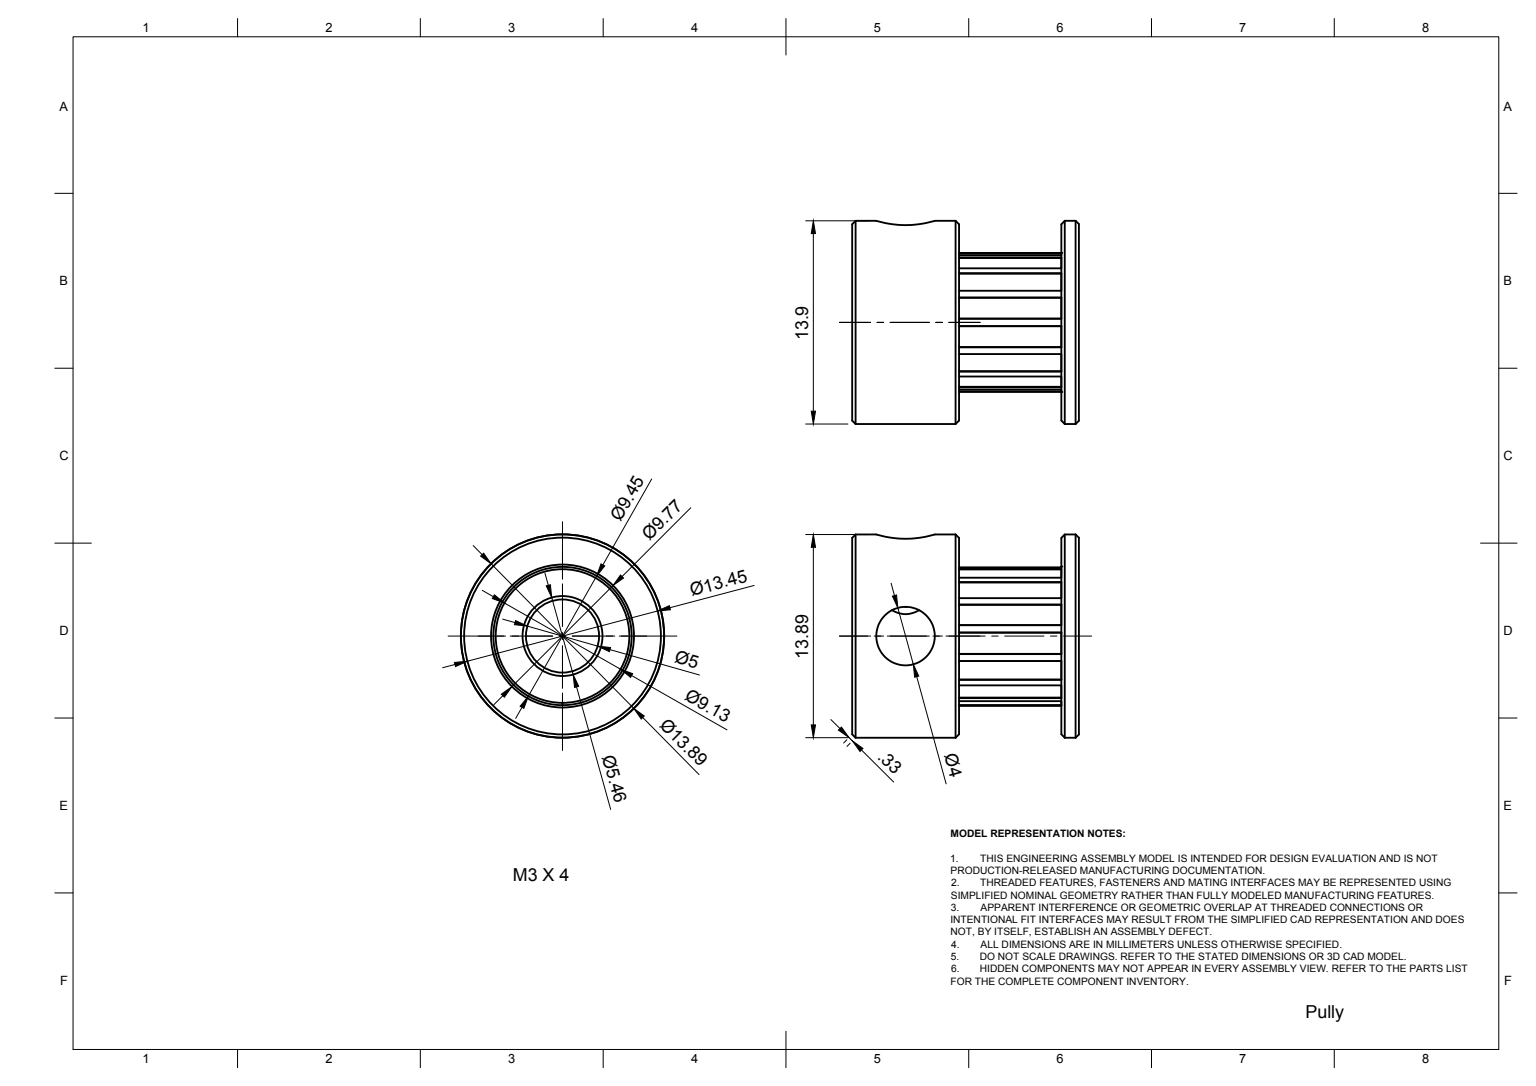
ISO-10303-21;
HEADER;
/* Generated by software containing ST-Developer
 * from STEP Tools, Inc. (www.steptools.com) 
 */

FILE_DESCRIPTION(
/* description */ (''),
/* implementation_level */ '2;1');

FILE_NAME(
/* name */ 'Pully.step',
/* time_stamp */ '2026-10-05T21:25:27-07:00',
/* author */ (''),
/* organization */ (''),
/* preprocessor_version */ 'ST-DEVELOPER v20.2',
/* originating_system */ 'Autodesk Translation Framework v15.15.0.0',
/* authorisation */ '');

FILE_SCHEMA (('AUTOMOTIVE_DESIGN { 1 0 10303 214 3 1 1 }'));
ENDSEC;

DATA;
#10=MECHANICAL_DESIGN_GEOMETRIC_PRESENTATION_REPRESENTATION('',(#33),#12118);
#27=SHAPE_REPRESENTATION_RELATIONSHIP('SRR','None',#12135,#30);
#30=ADVANCED_BREP_SHAPE_REPRESENTATION('',(#36),#12115);
#33=STYLED_ITEM('',(#12159),#36);
#36=MANIFOLD_SOLID_BREP('Body1',#2406);
#39=CONICAL_SURFACE('',#2637,6.82923606324244,0.788206310939685);
#40=CONICAL_SURFACE('',#2641,6.83201065632366,0.782590015855212);
#41=CONICAL_SURFACE('',#2645,4.80296382139185,0.926815431707518);
#42=CONICAL_SURFACE('',#2647,4.64521779108966,0.920500215637548);
#43=CONICAL_SURFACE('',#2651,2.61128051468949,0.789543103695558);
#44=CONICAL_SURFACE('',#2652,2.61559010295572,0.781253223099339);
#45=CONICAL_SURFACE('',#2656,4.64520588040018,0.911866720012535);
#46=CONICAL_SURFACE('',#2658,4.80503122320831,0.931803832862888);
#47=CONICAL_SURFACE('',#2662,6.83593993841137,0.77406839497658);
#48=CONICAL_SURFACE('',#2666,6.82905809599587,0.796727931818318);
#49=FACE_BOUND('',#442,.T.);
#50=FACE_BOUND('',#444,.T.);
#51=FACE_BOUND('',#447,.T.);
#52=FACE_BOUND('',#450,.T.);
#53=FACE_BOUND('',#454,.T.);
#54=FACE_BOUND('',#458,.T.);
#55=FACE_BOUND('',#462,.T.);
#58=PLANE('',#2453);
#59=PLANE('',#2464);
#60=PLANE('',#2475);
#61=PLANE('',#2486);
#62=PLANE('',#2497);
#63=PLANE('',#2508);
#64=PLANE('',#2519);
#65=PLANE('',#2530);
#66=PLANE('',#2541);
#67=PLANE('',#2552);
#68=PLANE('',#2563);
#69=PLANE('',#2574);
#70=PLANE('',#2585);
#71=PLANE('',#2596);
#72=PLANE('',#2626);
#73=PLANE('',#2633);
#74=PLANE('',#2635);
#75=PLANE('',#2643);
#76=PLANE('',#2649);
#77=PLANE('',#2654);
#78=PLANE('',#2660);
#97=CIRCLE('',#2447,2.50080065552765);
#98=CIRCLE('',#2448,2.50080065552765);
#99=CIRCLE('',#2451,0.124032861755453);
#100=CIRCLE('',#2452,0.124032861755453);
#101=CIRCLE('',#2454,4.75930776765241);
#102=CIRCLE('',#2455,0.749041401963156);
#103=CIRCLE('',#2456,0.124032861755453);
#104=CIRCLE('',#2458,0.749041401963156);
#105=CIRCLE('',#2460,0.124032861755453);
#106=CIRCLE('',#2462,0.124032861755453);
#107=CIRCLE('',#2463,0.124032861755453);
#108=CIRCLE('',#2465,4.75930776765241);
#109=CIRCLE('',#2466,0.749041401963156);
#110=CIRCLE('',#2467,0.124032861755453);
#111=CIRCLE('',#2469,0.749041401963156);
#112=CIRCLE('',#2471,0.124032861755453);
#113=CIRCLE('',#2473,0.124032861755453);
#114=CIRCLE('',#2474,0.124032861755453);
#115=CIRCLE('',#2476,4.75930776765241);
#116=CIRCLE('',#2477,0.749041401963155);
#117=CIRCLE('',#2478,0.124032861755453);
#118=CIRCLE('',#2480,0.749041401963155);
#119=CIRCLE('',#2482,0.124032861755453);
#120=CIRCLE('',#2484,0.124032861755453);
#121=CIRCLE('',#2485,0.124032861755453);
#122=CIRCLE('',#2487,4.75930776765241);
#123=CIRCLE('',#2488,0.749041401963156);
#124=CIRCLE('',#2489,0.124032861755453);
#125=CIRCLE('',#2491,0.749041401963156);
#126=CIRCLE('',#2493,0.124032861755453);
#127=CIRCLE('',#2495,0.124032861755453);
#128=CIRCLE('',#2496,0.124032861755453);
#129=CIRCLE('',#2498,4.75930776765241);
#130=CIRCLE('',#2499,0.749041401963155);
#131=CIRCLE('',#2500,0.124032861755453);
#132=CIRCLE('',#2502,0.749041401963155);
#133=CIRCLE('',#2504,0.124032861755453);
#134=CIRCLE('',#2506,0.124032861755453);
#135=CIRCLE('',#2507,0.124032861755453);
#136=CIRCLE('',#2509,4.75930776765241);
#137=CIRCLE('',#2510,0.749041401963156);
#138=CIRCLE('',#2511,0.124032861755453);
#139=CIRCLE('',#2513,0.749041401963156);
#140=CIRCLE('',#2515,0.124032861755453);
#141=CIRCLE('',#2517,0.124032861755453);
#142=CIRCLE('',#2518,0.124032861755453);
#143=CIRCLE('',#2520,4.75930776765241);
#144=CIRCLE('',#2521,0.749041401963155);
#145=CIRCLE('',#2522,0.124032861755453);
#146=CIRCLE('',#2524,0.749041401963155);
#147=CIRCLE('',#2526,0.124032861755453);
#148=CIRCLE('',#2528,0.124032861755453);
#149=CIRCLE('',#2529,0.124032861755453);
#150=CIRCLE('',#2531,4.75930776765241);
#151=CIRCLE('',#2532,0.749041401963156);
#152=CIRCLE('',#2533,0.124032861755453);
#153=CIRCLE('',#2535,0.749041401963156);
#154=CIRCLE('',#2537,0.124032861755453);
#155=CIRCLE('',#2539,0.124032861755453);
#156=CIRCLE('',#2540,0.124032861755453);
#157=CIRCLE('',#2542,4.75930776765241);
#158=CIRCLE('',#2543,0.749041401963155);
#159=CIRCLE('',#2544,0.124032861755453);
#160=CIRCLE('',#2546,0.749041401963155);
#161=CIRCLE('',#2548,0.124032861755453);
#162=CIRCLE('',#2550,0.124032861755453);
#163=CIRCLE('',#2551,0.124032861755453);
#164=CIRCLE('',#2553,4.75930776765241);
#165=CIRCLE('',#2554,0.749041401963156);
#166=CIRCLE('',#2555,0.124032861755453);
#167=CIRCLE('',#2557,0.749041401963156);
#168=CIRCLE('',#2559,0.124032861755453);
#169=CIRCLE('',#2561,0.124032861755453);
#170=CIRCLE('',#2562,0.124032861755453);
#171=CIRCLE('',#2564,4.75930776765241);
#172=CIRCLE('',#2565,0.749041401963156);
#173=CIRCLE('',#2566,0.124032861755453);
#174=CIRCLE('',#2568,0.749041401963156);
#175=CIRCLE('',#2570,0.124032861755453);
#176=CIRCLE('',#2572,0.124032861755453);
#177=CIRCLE('',#2573,0.124032861755453);
#178=CIRCLE('',#2575,4.75930776765241);
#179=CIRCLE('',#2576,0.749041401963155);
#180=CIRCLE('',#2577,0.124032861755453);
#181=CIRCLE('',#2579,0.749041401963155);
#182=CIRCLE('',#2581,0.124032861755453);
#183=CIRCLE('',#2583,0.124032861755453);
#184=CIRCLE('',#2584,0.124032861755453);
#185=CIRCLE('',#2586,4.75930776765241);
#186=CIRCLE('',#2587,0.749041401963156);
#187=CIRCLE('',#2588,0.124032861755453);
#188=CIRCLE('',#2590,0.749041401963156);
#189=CIRCLE('',#2592,0.124032861755453);
#190=CIRCLE('',#2594,0.124032861755453);
#191=CIRCLE('',#2595,0.124032861755453);
#192=CIRCLE('',#2597,4.75930776765241);
#193=CIRCLE('',#2598,0.749041401963155);
#194=CIRCLE('',#2599,0.124032861755453);
#195=CIRCLE('',#2601,0.749041401963155);
#196=CIRCLE('',#2603,0.124032861755453);
#197=CIRCLE('',#2605,4.75930776765241);
#198=CIRCLE('',#2606,4.75930776765241);
#199=CIRCLE('',#2607,4.75930776765241);
#200=CIRCLE('',#2608,4.75930776765241);
#201=CIRCLE('',#2609,4.75930776765241);
#202=CIRCLE('',#2610,4.75930776765241);
#203=CIRCLE('',#2611,4.75930776765241);
#204=CIRCLE('',#2612,4.75930776765241);
#205=CIRCLE('',#2613,4.75930776765241);
#206=CIRCLE('',#2614,4.75930776765241);
#207=CIRCLE('',#2615,4.75930776765241);
#208=CIRCLE('',#2616,4.75930776765241);
#209=CIRCLE('',#2617,4.75930776765241);
#210=CIRCLE('',#2618,4.75930776765241);
#211=CIRCLE('',#2619,4.75930776765241);
#212=CIRCLE('',#2620,4.75930776765241);
#213=CIRCLE('',#2621,4.75930776765241);
#214=CIRCLE('',#2622,4.75930776765241);
#215=CIRCLE('',#2624,0.124032861755453);
#216=CIRCLE('',#2625,0.124032861755453);
#217=CIRCLE('',#2627,0.749041401963155);
#218=CIRCLE('',#2628,0.124032861755453);
#219=CIRCLE('',#2630,0.749041401963155);
#220=CIRCLE('',#2632,0.124032861755453);
#221=CIRCLE('',#2634,6.71146155382814);
#222=CIRCLE('',#2636,6.71146155382814);
#223=CIRCLE('',#2638,6.94701057265674);
#224=CIRCLE('',#2640,6.94701057265674);
#225=CIRCLE('',#2642,6.71701073999059);
#226=CIRCLE('',#2644,4.88235460250674);
#227=CIRCLE('',#2646,4.72357304027696);
#228=CIRCLE('',#2648,4.56686254190236);
#229=CIRCLE('',#2650,2.72176037385134);
#230=CIRCLE('',#2653,2.7303795503838);
#231=CIRCLE('',#2655,4.56694754124435);
#232=CIRCLE('',#2657,4.72346421955602);
#233=CIRCLE('',#2659,4.8865982268606);
#234=CIRCLE('',#2661,6.72522523865914);
#235=CIRCLE('',#2663,6.94665463816359);
#236=CIRCLE('',#2665,6.94665463816359);
#245=FACE_OUTER_BOUND('',#377,.T.);
#246=FACE_OUTER_BOUND('',#378,.T.);
#247=FACE_OUTER_BOUND('',#379,.T.);
#248=FACE_OUTER_BOUND('',#380,.T.);
#249=FACE_OUTER_BOUND('',#381,.T.);
#250=FACE_OUTER_BOUND('',#382,.T.);
#251=FACE_OUTER_BOUND('',#383,.T.);
#252=FACE_OUTER_BOUND('',#384,.T.);
#253=FACE_OUTER_BOUND('',#385,.T.);
#254=FACE_OUTER_BOUND('',#386,.T.);
#255=FACE_OUTER_BOUND('',#387,.T.);
#256=FACE_OUTER_BOUND('',#388,.T.);
#257=FACE_OUTER_BOUND('',#389,.T.);
#258=FACE_OUTER_BOUND('',#390,.T.);
#259=FACE_OUTER_BOUND('',#391,.T.);
#260=FACE_OUTER_BOUND('',#392,.T.);
#261=FACE_OUTER_BOUND('',#393,.T.);
#262=FACE_OUTER_BOUND('',#394,.T.);
#263=FACE_OUTER_BOUND('',#395,.T.);
#264=FACE_OUTER_BOUND('',#396,.T.);
#265=FACE_OUTER_BOUND('',#397,.T.);
#266=FACE_OUTER_BOUND('',#398,.T.);
#267=FACE_OUTER_BOUND('',#399,.T.);
#268=FACE_OUTER_BOUND('',#400,.T.);
#269=FACE_OUTER_BOUND('',#401,.T.);
#270=FACE_OUTER_BOUND('',#402,.T.);
#271=FACE_OUTER_BOUND('',#403,.T.);
#272=FACE_OUTER_BOUND('',#404,.T.);
#273=FACE_OUTER_BOUND('',#405,.T.);
#274=FACE_OUTER_BOUND('',#406,.T.);
#275=FACE_OUTER_BOUND('',#407,.T.);
#276=FACE_OUTER_BOUND('',#408,.T.);
#277=FACE_OUTER_BOUND('',#409,.T.);
#278=FACE_OUTER_BOUND('',#410,.T.);
#279=FACE_OUTER_BOUND('',#411,.T.);
#280=FACE_OUTER_BOUND('',#412,.T.);
#281=FACE_OUTER_BOUND('',#413,.T.);
#282=FACE_OUTER_BOUND('',#414,.T.);
#283=FACE_OUTER_BOUND('',#415,.T.);
#284=FACE_OUTER_BOUND('',#416,.T.);
#285=FACE_OUTER_BOUND('',#417,.T.);
#286=FACE_OUTER_BOUND('',#418,.T.);
#287=FACE_OUTER_BOUND('',#419,.T.);
#288=FACE_OUTER_BOUND('',#420,.T.);
#289=FACE_OUTER_BOUND('',#421,.T.);
#290=FACE_OUTER_BOUND('',#422,.T.);
#291=FACE_OUTER_BOUND('',#423,.T.);
#292=FACE_OUTER_BOUND('',#424,.T.);
#293=FACE_OUTER_BOUND('',#425,.T.);
#294=FACE_OUTER_BOUND('',#426,.T.);
#295=FACE_OUTER_BOUND('',#427,.T.);
#296=FACE_OUTER_BOUND('',#428,.T.);
#297=FACE_OUTER_BOUND('',#429,.T.);
#298=FACE_OUTER_BOUND('',#430,.T.);
#299=FACE_OUTER_BOUND('',#431,.T.);
#300=FACE_OUTER_BOUND('',#432,.T.);
#301=FACE_OUTER_BOUND('',#433,.T.);
#302=FACE_OUTER_BOUND('',#434,.T.);
#303=FACE_OUTER_BOUND('',#435,.T.);
#304=FACE_OUTER_BOUND('',#436,.T.);
#305=FACE_OUTER_BOUND('',#437,.T.);
#306=FACE_OUTER_BOUND('',#438,.T.);
#307=FACE_OUTER_BOUND('',#439,.T.);
#308=FACE_OUTER_BOUND('',#440,.T.);
#309=FACE_OUTER_BOUND('',#441,.T.);
#310=FACE_OUTER_BOUND('',#443,.T.);
#311=FACE_OUTER_BOUND('',#445,.T.);
#312=FACE_OUTER_BOUND('',#446,.T.);
#313=FACE_OUTER_BOUND('',#448,.T.);
#314=FACE_OUTER_BOUND('',#449,.T.);
#315=FACE_OUTER_BOUND('',#451,.T.);
#316=FACE_OUTER_BOUND('',#452,.T.);
#317=FACE_OUTER_BOUND('',#453,.T.);
#318=FACE_OUTER_BOUND('',#455,.T.);
#319=FACE_OUTER_BOUND('',#456,.T.);
#320=FACE_OUTER_BOUND('',#457,.T.);
#321=FACE_OUTER_BOUND('',#459,.T.);
#322=FACE_OUTER_BOUND('',#460,.T.);
#323=FACE_OUTER_BOUND('',#461,.T.);
#324=FACE_OUTER_BOUND('',#463,.T.);
#325=FACE_OUTER_BOUND('',#464,.T.);
#326=FACE_OUTER_BOUND('',#465,.T.);
#377=EDGE_LOOP('',(#1471,#1472,#1473,#1474,#1475,#1476,#1477));
#378=EDGE_LOOP('',(#1478,#1479,#1480,#1481,#1482,#1483,#1484,#1485,#1486,
#1487,#1488,#1489));
#379=EDGE_LOOP('',(#1490,#1491,#1492,#1493,#1494,#1495,#1496,#1497,#1498,
#1499));
#380=EDGE_LOOP('',(#1500,#1501,#1502,#1503));
#381=EDGE_LOOP('',(#1504,#1505,#1506,#1507));
#382=EDGE_LOOP('',(#1508,#1509,#1510,#1511));
#383=EDGE_LOOP('',(#1512,#1513,#1514,#1515));
#384=EDGE_LOOP('',(#1516,#1517,#1518,#1519));
#385=EDGE_LOOP('',(#1520,#1521,#1522,#1523));
#386=EDGE_LOOP('',(#1524,#1525,#1526,#1527));
#387=EDGE_LOOP('',(#1528,#1529,#1530,#1531));
#388=EDGE_LOOP('',(#1532,#1533,#1534,#1535));
#389=EDGE_LOOP('',(#1536,#1537,#1538,#1539));
#390=EDGE_LOOP('',(#1540,#1541,#1542,#1543));
#391=EDGE_LOOP('',(#1544,#1545,#1546,#1547));
#392=EDGE_LOOP('',(#1548,#1549,#1550,#1551));
#393=EDGE_LOOP('',(#1552,#1553,#1554,#1555));
#394=EDGE_LOOP('',(#1556,#1557,#1558,#1559));
#395=EDGE_LOOP('',(#1560,#1561,#1562,#1563));
#396=EDGE_LOOP('',(#1564,#1565,#1566,#1567));
#397=EDGE_LOOP('',(#1568,#1569,#1570,#1571));
#398=EDGE_LOOP('',(#1572,#1573,#1574,#1575));
#399=EDGE_LOOP('',(#1576,#1577,#1578,#1579));
#400=EDGE_LOOP('',(#1580,#1581,#1582,#1583));
#401=EDGE_LOOP('',(#1584,#1585,#1586,#1587));
#402=EDGE_LOOP('',(#1588,#1589,#1590,#1591));
#403=EDGE_LOOP('',(#1592,#1593,#1594,#1595));
#404=EDGE_LOOP('',(#1596,#1597,#1598,#1599));
#405=EDGE_LOOP('',(#1600,#1601,#1602,#1603));
#406=EDGE_LOOP('',(#1604,#1605,#1606,#1607));
#407=EDGE_LOOP('',(#1608,#1609,#1610,#1611));
#408=EDGE_LOOP('',(#1612,#1613,#1614,#1615));
#409=EDGE_LOOP('',(#1616,#1617,#1618,#1619));
#410=EDGE_LOOP('',(#1620,#1621,#1622,#1623));
#411=EDGE_LOOP('',(#1624,#1625,#1626,#1627));
#412=EDGE_LOOP('',(#1628,#1629,#1630,#1631));
#413=EDGE_LOOP('',(#1632,#1633,#1634,#1635));
#414=EDGE_LOOP('',(#1636,#1637,#1638,#1639));
#415=EDGE_LOOP('',(#1640,#1641,#1642,#1643));
#416=EDGE_LOOP('',(#1644,#1645,#1646,#1647));
#417=EDGE_LOOP('',(#1648,#1649,#1650,#1651));
#418=EDGE_LOOP('',(#1652,#1653,#1654,#1655));
#419=EDGE_LOOP('',(#1656,#1657,#1658,#1659));
#420=EDGE_LOOP('',(#1660,#1661,#1662,#1663));
#421=EDGE_LOOP('',(#1664,#1665,#1666,#1667));
#422=EDGE_LOOP('',(#1668,#1669,#1670,#1671));
#423=EDGE_LOOP('',(#1672,#1673,#1674,#1675));
#424=EDGE_LOOP('',(#1676,#1677,#1678,#1679));
#425=EDGE_LOOP('',(#1680,#1681,#1682,#1683));
#426=EDGE_LOOP('',(#1684,#1685,#1686,#1687));
#427=EDGE_LOOP('',(#1688,#1689,#1690,#1691));
#428=EDGE_LOOP('',(#1692,#1693,#1694,#1695));
#429=EDGE_LOOP('',(#1696,#1697,#1698,#1699));
#430=EDGE_LOOP('',(#1700,#1701,#1702,#1703));
#431=EDGE_LOOP('',(#1704,#1705,#1706,#1707));
#432=EDGE_LOOP('',(#1708,#1709,#1710,#1711));
#433=EDGE_LOOP('',(#1712,#1713,#1714,#1715));
#434=EDGE_LOOP('',(#1716,#1717,#1718,#1719));
#435=EDGE_LOOP('',(#1720,#1721,#1722,#1723));
#436=EDGE_LOOP('',(#1724,#1725,#1726,#1727,#1728,#1729,#1730,#1731,#1732,
#1733,#1734,#1735,#1736,#1737,#1738,#1739,#1740,#1741,#1742,#1743,#1744,
#1745,#1746,#1747,#1748,#1749,#1750,#1751,#1752,#1753,#1754,#1755,#1756,
#1757,#1758,#1759,#1760,#1761,#1762,#1763,#1764,#1765,#1766,#1767,#1768,
#1769,#1770,#1771,#1772,#1773,#1774,#1775,#1776,#1777,#1778,#1779,#1780,
#1781,#1782,#1783,#1784,#1785,#1786,#1787));
#437=EDGE_LOOP('',(#1788,#1789,#1790,#1791));
#438=EDGE_LOOP('',(#1792,#1793,#1794,#1795,#1796));
#439=EDGE_LOOP('',(#1797,#1798,#1799,#1800));
#440=EDGE_LOOP('',(#1801,#1802,#1803,#1804));
#441=EDGE_LOOP('',(#1805));
#442=EDGE_LOOP('',(#1806));
#443=EDGE_LOOP('',(#1807));
#444=EDGE_LOOP('',(#1808,#1809,#1810,#1811,#1812,#1813,#1814,#1815,#1816,
#1817,#1818,#1819,#1820,#1821,#1822,#1823,#1824,#1825,#1826,#1827,#1828,
#1829,#1830,#1831,#1832,#1833,#1834,#1835,#1836,#1837,#1838,#1839,#1840,
#1841,#1842,#1843,#1844,#1845,#1846,#1847,#1848,#1849,#1850,#1851,#1852,
#1853,#1854,#1855,#1856,#1857,#1858,#1859,#1860,#1861,#1862,#1863,#1864,
#1865,#1866,#1867));
#445=EDGE_LOOP('',(#1868,#1869,#1870,#1871));
#446=EDGE_LOOP('',(#1872,#1873,#1874,#1875,#1876,#1877,#1878,#1879,#1880));
#447=EDGE_LOOP('',(#1881,#1882));
#448=EDGE_LOOP('',(#1883,#1884,#1885,#1886));
#449=EDGE_LOOP('',(#1887));
#450=EDGE_LOOP('',(#1888));
#451=EDGE_LOOP('',(#1889,#1890,#1891,#1892));
#452=EDGE_LOOP('',(#1893,#1894,#1895,#1896));
#453=EDGE_LOOP('',(#1897));
#454=EDGE_LOOP('',(#1898));
#455=EDGE_LOOP('',(#1899,#1900,#1901,#1902));
#456=EDGE_LOOP('',(#1903,#1904,#1905,#1906));
#457=EDGE_LOOP('',(#1907));
#458=EDGE_LOOP('',(#1908));
#459=EDGE_LOOP('',(#1909,#1910,#1911,#1912));
#460=EDGE_LOOP('',(#1913,#1914,#1915,#1916));
#461=EDGE_LOOP('',(#1917));
#462=EDGE_LOOP('',(#1918));
#463=EDGE_LOOP('',(#1919,#1920,#1921,#1922));
#464=EDGE_LOOP('',(#1923,#1924,#1925,#1926));
#465=EDGE_LOOP('',(#1927,#1928,#1929,#1930));
#518=LINE('',#3487,#656);
#519=LINE('',#3529,#657);
#520=LINE('',#3557,#658);
#521=LINE('',#3577,#659);
#522=LINE('',#3621,#660);
#523=LINE('',#3625,#661);
#524=LINE('',#3636,#662);
#525=LINE('',#3639,#663);
#526=LINE('',#3644,#664);
#527=LINE('',#3648,#665);
#528=LINE('',#3659,#666);
#529=LINE('',#3662,#667);
#530=LINE('',#3667,#668);
#531=LINE('',#3671,#669);
#532=LINE('',#3682,#670);
#533=LINE('',#3685,#671);
#534=LINE('',#3690,#672);
#535=LINE('',#3694,#673);
#536=LINE('',#3705,#674);
#537=LINE('',#3708,#675);
#538=LINE('',#3713,#676);
#539=LINE('',#3717,#677);
#540=LINE('',#3728,#678);
#541=LINE('',#3731,#679);
#542=LINE('',#3736,#680);
#543=LINE('',#3740,#681);
#544=LINE('',#3751,#682);
#545=LINE('',#3754,#683);
#546=LINE('',#3759,#684);
#547=LINE('',#3763,#685);
#548=LINE('',#3774,#686);
#549=LINE('',#3777,#687);
#550=LINE('',#3782,#688);
#551=LINE('',#3786,#689);
#552=LINE('',#3797,#690);
#553=LINE('',#3800,#691);
#554=LINE('',#3805,#692);
#555=LINE('',#3809,#693);
#556=LINE('',#3820,#694);
#557=LINE('',#3823,#695);
#558=LINE('',#3828,#696);
#559=LINE('',#3832,#697);
#560=LINE('',#3843,#698);
#561=LINE('',#3846,#699);
#562=LINE('',#3851,#700);
#563=LINE('',#3855,#701);
#564=LINE('',#3866,#702);
#565=LINE('',#3869,#703);
#566=LINE('',#3874,#704);
#567=LINE('',#3878,#705);
#568=LINE('',#3889,#706);
#569=LINE('',#3892,#707);
#570=LINE('',#3897,#708);
#571=LINE('',#3901,#709);
#572=LINE('',#3912,#710);
#573=LINE('',#3915,#711);
#574=LINE('',#3920,#712);
#575=LINE('',#3924,#713);
#576=LINE('',#3935,#714);
#577=LINE('',#3938,#715);
#578=LINE('',#3945,#716);
#579=LINE('',#3950,#717);
#580=LINE('',#3967,#718);
#581=LINE('',#3972,#719);
#582=LINE('',#3981,#720);
#583=LINE('',#3993,#721);
#584=LINE('',#3997,#722);
#585=LINE('',#3998,#723);
#586=LINE('',#4001,#724);
#587=LINE('',#4009,#725);
#588=LINE('',#4012,#726);
#589=LINE('',#4018,#727);
#590=LINE('',#4021,#728);
#591=LINE('',#4029,#729);
#592=LINE('',#4032,#730);
#593=LINE('',#4040,#731);
#594=LINE('',#4044,#732);
#595=LINE('',#4046,#733);
#656=VECTOR('',#2732,2.00054127207588);
#657=VECTOR('',#2737,2.50080065552765);
#658=VECTOR('',#2738,2.50080065552765);
#659=VECTOR('',#2743,2.00007126058529);
#660=VECTOR('',#2746,10.);
#661=VECTOR('',#2749,10.);
#662=VECTOR('',#2764,10.);
#663=VECTOR('',#2767,10.);
#664=VECTOR('',#2772,10.);
#665=VECTOR('',#2775,10.);
#666=VECTOR('',#2790,10.);
#667=VECTOR('',#2793,10.);
#668=VECTOR('',#2798,10.);
#669=VECTOR('',#2801,10.);
#670=VECTOR('',#2816,10.);
#671=VECTOR('',#2819,10.);
#672=VECTOR('',#2824,10.);
#673=VECTOR('',#2827,10.);
#674=VECTOR('',#2842,10.);
#675=VECTOR('',#2845,10.);
#676=VECTOR('',#2850,10.);
#677=VECTOR('',#2853,10.);
#678=VECTOR('',#2868,10.);
#679=VECTOR('',#2871,10.);
#680=VECTOR('',#2876,10.);
#681=VECTOR('',#2879,10.);
#682=VECTOR('',#2894,10.);
#683=VECTOR('',#2897,10.);
#684=VECTOR('',#2902,10.);
#685=VECTOR('',#2905,10.);
#686=VECTOR('',#2920,10.);
#687=VECTOR('',#2923,10.);
#688=VECTOR('',#2928,10.);
#689=VECTOR('',#2931,10.);
#690=VECTOR('',#2946,10.);
#691=VECTOR('',#2949,10.);
#692=VECTOR('',#2954,10.);
#693=VECTOR('',#2957,10.);
#694=VECTOR('',#2972,10.);
#695=VECTOR('',#2975,10.);
#696=VECTOR('',#2980,10.);
#697=VECTOR('',#2983,10.);
#698=VECTOR('',#2998,10.);
#699=VECTOR('',#3001,10.);
#700=VECTOR('',#3006,10.);
#701=VECTOR('',#3009,10.);
#702=VECTOR('',#3024,10.);
#703=VECTOR('',#3027,10.);
#704=VECTOR('',#3032,10.);
#705=VECTOR('',#3035,10.);
#706=VECTOR('',#3050,10.);
#707=VECTOR('',#3053,10.);
#708=VECTOR('',#3058,10.);
#709=VECTOR('',#3061,10.);
#710=VECTOR('',#3076,10.);
#711=VECTOR('',#3079,10.);
#712=VECTOR('',#3084,10.);
#713=VECTOR('',#3087,10.);
#714=VECTOR('',#3102,10.);
#715=VECTOR('',#3105,10.);
#716=VECTOR('',#3112,4.75930776765241);
#717=VECTOR('',#3117,10.);
#718=VECTOR('',#3148,10.);
#719=VECTOR('',#3153,10.);
#720=VECTOR('',#3166,10.);
#721=VECTOR('',#3183,6.82923606324244);
#722=VECTOR('',#3188,6.94701057265674);
#723=VECTOR('',#3189,6.94701057265674);
#724=VECTOR('',#3192,6.83201065632366);
#725=VECTOR('',#3203,4.80296382139185);
#726=VECTOR('',#3206,4.64521779108966);
#727=VECTOR('',#3215,2.61128051468949);
#728=VECTOR('',#3218,2.61559010295572);
#729=VECTOR('',#3229,4.64520588040018);
#730=VECTOR('',#3232,4.80503122320831);
#731=VECTOR('',#3243,6.83593993841137);
#732=VECTOR('',#3248,6.94665463816359);
#733=VECTOR('',#3251,6.82905809599587);
#794=B_SPLINE_CURVE_WITH_KNOTS('',3,(#3435,#3436,#3437,#3438,#3439,#3440,
#3441,#3442,#3443,#3444,#3445,#3446,#3447,#3448,#3449,#3450,#3451,#3452),
 .UNSPECIFIED.,.F.,.F.,(4,2,2,2,2,2,2,2,4),(-1.19269999759714,-1.12829413515979,
-1.04879502724507,-0.969295919330357,-0.889796811415643,-0.81029770350093,
-0.728247491527251,-0.687222385540411,-0.646197279553572),.UNSPECIFIED.);
#795=B_SPLINE_CURVE_WITH_KNOTS('',3,(#3454,#3455,#3456,#3457,#3458,#3459,
#3460,#3461,#3462,#3463,#3464,#3465,#3466,#3467),.UNSPECIFIED.,.F.,.F.,
(4,2,2,2,2,2,4),(-0.499257003558056,-0.483639998022121,-0.442252990706973,
-0.400865983391825,-0.359481492928847,-0.318097002465869,-0.302466663278823),
 .UNSPECIFIED.);
#796=B_SPLINE_CURVE_WITH_KNOTS('',3,(#3468,#3469,#3470,#3471,#3472,#3473,
#3474,#3475,#3476,#3477,#3478,#3479,#3480,#3481,#3482,#3483,#3484,#3485),
 .UNSPECIFIED.,.F.,.F.,(4,2,2,2,2,2,2,2,4),(-0.646197279553572,-0.605172173566732,
-0.564147067579893,-0.482096855606214,-0.4025977476915,-0.323098639776786,
-0.243599531862072,-0.164100423947358,-0.0997053765976701),
 .UNSPECIFIED.);
#797=B_SPLINE_CURVE_WITH_KNOTS('',3,(#3489,#3490,#3491,#3492,#3493,#3494,
#3495,#3496,#3497,#3498,#3499,#3500,#3501,#3502,#3503,#3504,#3505,#3506),
 .UNSPECIFIED.,.F.,.F.,(4,2,2,2,2,2,2,2,4),(0.,0.0758326534165654,0.151665306833131,
0.227478914786725,0.303292522740319,0.379106130693913,0.454919738647507,
0.530752392064072,0.606585045480638),.UNSPECIFIED.);
#798=B_SPLINE_CURVE_WITH_KNOTS('',3,(#3507,#3508,#3509,#3510,#3511,#3512,
#3513,#3514,#3515,#3516,#3517,#3518,#3519,#3520,#3521,#3522,#3523,#3524),
 .UNSPECIFIED.,.F.,.F.,(4,2,2,2,2,2,2,2,4),(0.606585045480638,0.682417698897203,
0.758250352313769,0.834063960267363,0.909877568220957,0.985691176174551,
1.06150478412814,1.13733743754471,1.21317009096128),.UNSPECIFIED.);
#799=B_SPLINE_CURVE_WITH_KNOTS('',3,(#3531,#3532,#3533,#3534,#3535,#3536,
#3537,#3538,#3539,#3540,#3541,#3542),.UNSPECIFIED.,.F.,.F.,(4,2,2,2,2,4),
(0.969015815726938,1.04849387615309,1.12797193657924,1.20999651210758,1.25100879987175,
1.29202108763592),.UNSPECIFIED.);
#800=B_SPLINE_CURVE_WITH_KNOTS('',3,(#3544,#3545,#3546,#3547,#3548,#3549,
#3550,#3551,#3552,#3553,#3554,#3555),.UNSPECIFIED.,.F.,.F.,(4,2,2,2,2,4),
(1.29202108763592,1.33303337540009,1.37404566316426,1.45607023869259,1.53554829911875,
1.6150263595449),.UNSPECIFIED.);
#801=B_SPLINE_CURVE_WITH_KNOTS('',3,(#3559,#3560,#3561,#3562,#3563,#3564,
#3565,#3566),.UNSPECIFIED.,.F.,.F.,(4,2,2,4),(1.6150263595449,1.69450441997105,
1.7739824803972,1.83833088236406),.UNSPECIFIED.);
#802=B_SPLINE_CURVE_WITH_KNOTS('',3,(#3567,#3568,#3569,#3570,#3571,#3572,
#3573,#3574),.UNSPECIFIED.,.F.,.F.,(4,2,2,4),(0.745700478002982,0.810059694874633,
0.889537755300786,0.969015815726938),.UNSPECIFIED.);
#803=B_SPLINE_CURVE_WITH_KNOTS('',3,(#3579,#3580,#3581,#3582,#3583,#3584,
#3585,#3586,#3587,#3588),.UNSPECIFIED.,.F.,.F.,(4,2,2,2,4),(0.909661063924676,
0.985456641432266,1.06125221893986,1.13706681875305,1.21288141856623),
 .UNSPECIFIED.);
#804=B_SPLINE_CURVE_WITH_KNOTS('',3,(#3590,#3591,#3592,#3593,#3594,#3595,
#3596,#3597,#3598,#3599,#3600,#3601,#3602,#3603,#3604,#3605,#3606,#3607),
 .UNSPECIFIED.,.F.,.F.,(4,2,2,2,2,2,2,2,4),(0.303220354641559,0.379015932149148,
0.454811509656738,0.530626109469928,0.606440709283118,0.682255309096307,
0.758069908909497,0.833865486417087,0.909661063924676),.UNSPECIFIED.);
#805=B_SPLINE_CURVE_WITH_KNOTS('',3,(#3608,#3609,#3610,#3611,#3612,#3613,
#3614,#3615,#3616,#3617),.UNSPECIFIED.,.F.,.F.,(4,2,2,2,4),(1.21288141856623,
1.28869601837942,1.36451061819261,1.4403061957002,1.51610177320779),
 .UNSPECIFIED.);
#870=VERTEX_POINT('',#3433);
#871=VERTEX_POINT('',#3434);
#872=VERTEX_POINT('',#3453);
#873=VERTEX_POINT('',#3486);
#874=VERTEX_POINT('',#3488);
#875=VERTEX_POINT('',#3526);
#876=VERTEX_POINT('',#3528);
#877=VERTEX_POINT('',#3530);
#878=VERTEX_POINT('',#3543);
#879=VERTEX_POINT('',#3556);
#880=VERTEX_POINT('',#3576);
#881=VERTEX_POINT('',#3578);
#882=VERTEX_POINT('',#3589);
#883=VERTEX_POINT('',#3619);
#884=VERTEX_POINT('',#3620);
#885=VERTEX_POINT('',#3622);
#886=VERTEX_POINT('',#3624);
#887=VERTEX_POINT('',#3628);
#888=VERTEX_POINT('',#3630);
#889=VERTEX_POINT('',#3634);
#890=VERTEX_POINT('',#3638);
#891=VERTEX_POINT('',#3642);
#892=VERTEX_POINT('',#3643);
#893=VERTEX_POINT('',#3645);
#894=VERTEX_POINT('',#3647);
#895=VERTEX_POINT('',#3651);
#896=VERTEX_POINT('',#3653);
#897=VERTEX_POINT('',#3657);
#898=VERTEX_POINT('',#3661);
#899=VERTEX_POINT('',#3665);
#900=VERTEX_POINT('',#3666);
#901=VERTEX_POINT('',#3668);
#902=VERTEX_POINT('',#3670);
#903=VERTEX_POINT('',#3674);
#904=VERTEX_POINT('',#3676);
#905=VERTEX_POINT('',#3680);
#906=VERTEX_POINT('',#3684);
#907=VERTEX_POINT('',#3688);
#908=VERTEX_POINT('',#3689);
#909=VERTEX_POINT('',#3691);
#910=VERTEX_POINT('',#3693);
#911=VERTEX_POINT('',#3697);
#912=VERTEX_POINT('',#3699);
#913=VERTEX_POINT('',#3703);
#914=VERTEX_POINT('',#3707);
#915=VERTEX_POINT('',#3711);
#916=VERTEX_POINT('',#3712);
#917=VERTEX_POINT('',#3714);
#918=VERTEX_POINT('',#3716);
#919=VERTEX_POINT('',#3720);
#920=VERTEX_POINT('',#3722);
#921=VERTEX_POINT('',#3726);
#922=VERTEX_POINT('',#3730);
#923=VERTEX_POINT('',#3734);
#924=VERTEX_POINT('',#3735);
#925=VERTEX_POINT('',#3737);
#926=VERTEX_POINT('',#3739);
#927=VERTEX_POINT('',#3743);
#928=VERTEX_POINT('',#3745);
#929=VERTEX_POINT('',#3749);
#930=VERTEX_POINT('',#3753);
#931=VERTEX_POINT('',#3757);
#932=VERTEX_POINT('',#3758);
#933=VERTEX_POINT('',#3760);
#934=VERTEX_POINT('',#3762);
#935=VERTEX_POINT('',#3766);
#936=VERTEX_POINT('',#3768);
#937=VERTEX_POINT('',#3772);
#938=VERTEX_POINT('',#3776);
#939=VERTEX_POINT('',#3780);
#940=VERTEX_POINT('',#3781);
#941=VERTEX_POINT('',#3783);
#942=VERTEX_POINT('',#3785);
#943=VERTEX_POINT('',#3789);
#944=VERTEX_POINT('',#3791);
#945=VERTEX_POINT('',#3795);
#946=VERTEX_POINT('',#3799);
#947=VERTEX_POINT('',#3803);
#948=VERTEX_POINT('',#3804);
#949=VERTEX_POINT('',#3806);
#950=VERTEX_POINT('',#3808);
#951=VERTEX_POINT('',#3812);
#952=VERTEX_POINT('',#3814);
#953=VERTEX_POINT('',#3818);
#954=VERTEX_POINT('',#3822);
#955=VERTEX_POINT('',#3826);
#956=VERTEX_POINT('',#3827);
#957=VERTEX_POINT('',#3829);
#958=VERTEX_POINT('',#3831);
#959=VERTEX_POINT('',#3835);
#960=VERTEX_POINT('',#3837);
#961=VERTEX_POINT('',#3841);
#962=VERTEX_POINT('',#3845);
#963=VERTEX_POINT('',#3849);
#964=VERTEX_POINT('',#3850);
#965=VERTEX_POINT('',#3852);
#966=VERTEX_POINT('',#3854);
#967=VERTEX_POINT('',#3858);
#968=VERTEX_POINT('',#3860);
#969=VERTEX_POINT('',#3864);
#970=VERTEX_POINT('',#3868);
#971=VERTEX_POINT('',#3872);
#972=VERTEX_POINT('',#3873);
#973=VERTEX_POINT('',#3875);
#974=VERTEX_POINT('',#3877);
#975=VERTEX_POINT('',#3881);
#976=VERTEX_POINT('',#3883);
#977=VERTEX_POINT('',#3887);
#978=VERTEX_POINT('',#3891);
#979=VERTEX_POINT('',#3895);
#980=VERTEX_POINT('',#3896);
#981=VERTEX_POINT('',#3898);
#982=VERTEX_POINT('',#3900);
#983=VERTEX_POINT('',#3904);
#984=VERTEX_POINT('',#3906);
#985=VERTEX_POINT('',#3910);
#986=VERTEX_POINT('',#3914);
#987=VERTEX_POINT('',#3918);
#988=VERTEX_POINT('',#3919);
#989=VERTEX_POINT('',#3921);
#990=VERTEX_POINT('',#3923);
#991=VERTEX_POINT('',#3927);
#992=VERTEX_POINT('',#3929);
#993=VERTEX_POINT('',#3933);
#994=VERTEX_POINT('',#3937);
#995=VERTEX_POINT('',#3941);
#996=VERTEX_POINT('',#3942);
#997=VERTEX_POINT('',#3944);
#998=VERTEX_POINT('',#3947);
#999=VERTEX_POINT('',#3949);
#1000=VERTEX_POINT('',#3965);
#1001=VERTEX_POINT('',#3969);
#1002=VERTEX_POINT('',#3971);
#1003=VERTEX_POINT('',#3975);
#1004=VERTEX_POINT('',#3979);
#1005=VERTEX_POINT('',#3985);
#1006=VERTEX_POINT('',#3988);
#1007=VERTEX_POINT('',#3991);
#1008=VERTEX_POINT('',#3995);
#1009=VERTEX_POINT('',#4000);
#1010=VERTEX_POINT('',#4004);
#1011=VERTEX_POINT('',#4007);
#1012=VERTEX_POINT('',#4011);
#1013=VERTEX_POINT('',#4015);
#1014=VERTEX_POINT('',#4020);
#1015=VERTEX_POINT('',#4024);
#1016=VERTEX_POINT('',#4027);
#1017=VERTEX_POINT('',#4031);
#1018=VERTEX_POINT('',#4035);
#1019=VERTEX_POINT('',#4038);
#1020=VERTEX_POINT('',#4042);
#1109=EDGE_CURVE('',#870,#871,#794,.T.);
#1110=EDGE_CURVE('',#872,#870,#795,.T.);
#1111=EDGE_CURVE('',#871,#872,#796,.T.);
#1112=EDGE_CURVE('',#871,#873,#518,.T.);
#1113=EDGE_CURVE('',#874,#873,#797,.T.);
#1114=EDGE_CURVE('',#873,#874,#798,.T.);
#1115=EDGE_CURVE('',#875,#875,#97,.T.);
#1116=EDGE_CURVE('',#875,#876,#519,.T.);
#1117=EDGE_CURVE('',#876,#877,#799,.T.);
#1118=EDGE_CURVE('',#877,#878,#800,.T.);
#1119=EDGE_CURVE('',#878,#879,#520,.T.);
#1120=EDGE_CURVE('',#879,#879,#98,.T.);
#1121=EDGE_CURVE('',#878,#870,#801,.T.);
#1122=EDGE_CURVE('',#872,#876,#802,.T.);
#1123=EDGE_CURVE('',#877,#880,#521,.T.);
#1124=EDGE_CURVE('',#881,#880,#803,.T.);
#1125=EDGE_CURVE('',#882,#881,#804,.T.);
#1126=EDGE_CURVE('',#880,#882,#805,.T.);
#1127=EDGE_CURVE('',#883,#884,#522,.T.);
#1128=EDGE_CURVE('',#883,#885,#99,.T.);
#1129=EDGE_CURVE('',#885,#886,#523,.T.);
#1130=EDGE_CURVE('',#886,#884,#100,.T.);
#1131=EDGE_CURVE('',#884,#887,#101,.T.);
#1132=EDGE_CURVE('',#888,#886,#102,.T.);
#1133=EDGE_CURVE('',#887,#888,#103,.T.);
#1134=EDGE_CURVE('',#889,#885,#104,.T.);
#1135=EDGE_CURVE('',#889,#888,#524,.T.);
#1136=EDGE_CURVE('',#887,#890,#525,.T.);
#1137=EDGE_CURVE('',#889,#890,#105,.T.);
#1138=EDGE_CURVE('',#891,#892,#526,.T.);
#1139=EDGE_CURVE('',#891,#893,#106,.T.);
#1140=EDGE_CURVE('',#893,#894,#527,.T.);
#1141=EDGE_CURVE('',#894,#892,#107,.T.);
#1142=EDGE_CURVE('',#892,#895,#108,.T.);
#1143=EDGE_CURVE('',#896,#894,#109,.T.);
#1144=EDGE_CURVE('',#895,#896,#110,.T.);
#1145=EDGE_CURVE('',#897,#893,#111,.T.);
#1146=EDGE_CURVE('',#897,#896,#528,.T.);
#1147=EDGE_CURVE('',#895,#898,#529,.T.);
#1148=EDGE_CURVE('',#897,#898,#112,.T.);
#1149=EDGE_CURVE('',#899,#900,#530,.T.);
#1150=EDGE_CURVE('',#899,#901,#113,.T.);
#1151=EDGE_CURVE('',#901,#902,#531,.T.);
#1152=EDGE_CURVE('',#902,#900,#114,.T.);
#1153=EDGE_CURVE('',#900,#903,#115,.T.);
#1154=EDGE_CURVE('',#904,#902,#116,.T.);
#1155=EDGE_CURVE('',#903,#904,#117,.T.);
#1156=EDGE_CURVE('',#905,#901,#118,.T.);
#1157=EDGE_CURVE('',#905,#904,#532,.T.);
#1158=EDGE_CURVE('',#903,#906,#533,.T.);
#1159=EDGE_CURVE('',#905,#906,#119,.T.);
#1160=EDGE_CURVE('',#907,#908,#534,.T.);
#1161=EDGE_CURVE('',#907,#909,#120,.T.);
#1162=EDGE_CURVE('',#909,#910,#535,.T.);
#1163=EDGE_CURVE('',#910,#908,#121,.T.);
#1164=EDGE_CURVE('',#908,#911,#122,.T.);
#1165=EDGE_CURVE('',#912,#910,#123,.T.);
#1166=EDGE_CURVE('',#911,#912,#124,.T.);
#1167=EDGE_CURVE('',#913,#909,#125,.T.);
#1168=EDGE_CURVE('',#913,#912,#536,.T.);
#1169=EDGE_CURVE('',#911,#914,#537,.T.);
#1170=EDGE_CURVE('',#913,#914,#126,.T.);
#1171=EDGE_CURVE('',#915,#916,#538,.T.);
#1172=EDGE_CURVE('',#915,#917,#127,.T.);
#1173=EDGE_CURVE('',#917,#918,#539,.T.);
#1174=EDGE_CURVE('',#918,#916,#128,.T.);
#1175=EDGE_CURVE('',#916,#919,#129,.T.);
#1176=EDGE_CURVE('',#920,#918,#130,.T.);
#1177=EDGE_CURVE('',#919,#920,#131,.T.);
#1178=EDGE_CURVE('',#921,#917,#132,.T.);
#1179=EDGE_CURVE('',#921,#920,#540,.T.);
#1180=EDGE_CURVE('',#919,#922,#541,.T.);
#1181=EDGE_CURVE('',#921,#922,#133,.T.);
#1182=EDGE_CURVE('',#923,#924,#542,.T.);
#1183=EDGE_CURVE('',#923,#925,#134,.T.);
#1184=EDGE_CURVE('',#925,#926,#543,.T.);
#1185=EDGE_CURVE('',#926,#924,#135,.T.);
#1186=EDGE_CURVE('',#924,#927,#136,.T.);
#1187=EDGE_CURVE('',#928,#926,#137,.T.);
#1188=EDGE_CURVE('',#927,#928,#138,.T.);
#1189=EDGE_CURVE('',#929,#925,#139,.T.);
#1190=EDGE_CURVE('',#929,#928,#544,.T.);
#1191=EDGE_CURVE('',#927,#930,#545,.T.);
#1192=EDGE_CURVE('',#929,#930,#140,.T.);
#1193=EDGE_CURVE('',#931,#932,#546,.T.);
#1194=EDGE_CURVE('',#931,#933,#141,.T.);
#1195=EDGE_CURVE('',#933,#934,#547,.T.);
#1196=EDGE_CURVE('',#934,#932,#142,.T.);
#1197=EDGE_CURVE('',#932,#935,#143,.T.);
#1198=EDGE_CURVE('',#936,#934,#144,.T.);
#1199=EDGE_CURVE('',#935,#936,#145,.T.);
#1200=EDGE_CURVE('',#937,#933,#146,.T.);
#1201=EDGE_CURVE('',#937,#936,#548,.T.);
#1202=EDGE_CURVE('',#935,#938,#549,.T.);
#1203=EDGE_CURVE('',#937,#938,#147,.T.);
#1204=EDGE_CURVE('',#939,#940,#550,.T.);
#1205=EDGE_CURVE('',#939,#941,#148,.T.);
#1206=EDGE_CURVE('',#941,#942,#551,.T.);
#1207=EDGE_CURVE('',#942,#940,#149,.T.);
#1208=EDGE_CURVE('',#940,#943,#150,.T.);
#1209=EDGE_CURVE('',#944,#942,#151,.T.);
#1210=EDGE_CURVE('',#943,#944,#152,.T.);
#1211=EDGE_CURVE('',#945,#941,#153,.T.);
#1212=EDGE_CURVE('',#945,#944,#552,.T.);
#1213=EDGE_CURVE('',#943,#946,#553,.T.);
#1214=EDGE_CURVE('',#945,#946,#154,.T.);
#1215=EDGE_CURVE('',#947,#948,#554,.T.);
#1216=EDGE_CURVE('',#947,#949,#155,.T.);
#1217=EDGE_CURVE('',#949,#950,#555,.T.);
#1218=EDGE_CURVE('',#950,#948,#156,.T.);
#1219=EDGE_CURVE('',#948,#951,#157,.T.);
#1220=EDGE_CURVE('',#952,#950,#158,.T.);
#1221=EDGE_CURVE('',#951,#952,#159,.T.);
#1222=EDGE_CURVE('',#953,#949,#160,.T.);
#1223=EDGE_CURVE('',#953,#952,#556,.T.);
#1224=EDGE_CURVE('',#951,#954,#557,.T.);
#1225=EDGE_CURVE('',#953,#954,#161,.T.);
#1226=EDGE_CURVE('',#955,#956,#558,.T.);
#1227=EDGE_CURVE('',#955,#957,#162,.T.);
#1228=EDGE_CURVE('',#957,#958,#559,.T.);
#1229=EDGE_CURVE('',#958,#956,#163,.T.);
#1230=EDGE_CURVE('',#956,#959,#164,.T.);
#1231=EDGE_CURVE('',#960,#958,#165,.T.);
#1232=EDGE_CURVE('',#959,#960,#166,.T.);
#1233=EDGE_CURVE('',#961,#957,#167,.T.);
#1234=EDGE_CURVE('',#961,#960,#560,.T.);
#1235=EDGE_CURVE('',#959,#962,#561,.T.);
#1236=EDGE_CURVE('',#961,#962,#168,.T.);
#1237=EDGE_CURVE('',#963,#964,#562,.T.);
#1238=EDGE_CURVE('',#963,#965,#169,.T.);
#1239=EDGE_CURVE('',#965,#966,#563,.T.);
#1240=EDGE_CURVE('',#966,#964,#170,.T.);
#1241=EDGE_CURVE('',#964,#967,#171,.T.);
#1242=EDGE_CURVE('',#968,#966,#172,.T.);
#1243=EDGE_CURVE('',#967,#968,#173,.T.);
#1244=EDGE_CURVE('',#969,#965,#174,.T.);
#1245=EDGE_CURVE('',#969,#968,#564,.T.);
#1246=EDGE_CURVE('',#967,#970,#565,.T.);
#1247=EDGE_CURVE('',#969,#970,#175,.T.);
#1248=EDGE_CURVE('',#971,#972,#566,.T.);
#1249=EDGE_CURVE('',#971,#973,#176,.T.);
#1250=EDGE_CURVE('',#973,#974,#567,.T.);
#1251=EDGE_CURVE('',#974,#972,#177,.T.);
#1252=EDGE_CURVE('',#972,#975,#178,.T.);
#1253=EDGE_CURVE('',#976,#974,#179,.T.);
#1254=EDGE_CURVE('',#975,#976,#180,.T.);
#1255=EDGE_CURVE('',#977,#973,#181,.T.);
#1256=EDGE_CURVE('',#977,#976,#568,.T.);
#1257=EDGE_CURVE('',#975,#978,#569,.T.);
#1258=EDGE_CURVE('',#977,#978,#182,.T.);
#1259=EDGE_CURVE('',#979,#980,#570,.T.);
#1260=EDGE_CURVE('',#979,#981,#183,.T.);
#1261=EDGE_CURVE('',#981,#982,#571,.T.);
#1262=EDGE_CURVE('',#982,#980,#184,.T.);
#1263=EDGE_CURVE('',#980,#983,#185,.T.);
#1264=EDGE_CURVE('',#984,#982,#186,.T.);
#1265=EDGE_CURVE('',#983,#984,#187,.T.);
#1266=EDGE_CURVE('',#985,#981,#188,.T.);
#1267=EDGE_CURVE('',#985,#984,#572,.T.);
#1268=EDGE_CURVE('',#983,#986,#573,.T.);
#1269=EDGE_CURVE('',#985,#986,#189,.T.);
#1270=EDGE_CURVE('',#987,#988,#574,.T.);
#1271=EDGE_CURVE('',#987,#989,#190,.T.);
#1272=EDGE_CURVE('',#989,#990,#575,.T.);
#1273=EDGE_CURVE('',#990,#988,#191,.T.);
#1274=EDGE_CURVE('',#988,#991,#192,.T.);
#1275=EDGE_CURVE('',#992,#990,#193,.T.);
#1276=EDGE_CURVE('',#991,#992,#194,.T.);
#1277=EDGE_CURVE('',#993,#989,#195,.T.);
#1278=EDGE_CURVE('',#993,#992,#576,.T.);
#1279=EDGE_CURVE('',#991,#994,#577,.T.);
#1280=EDGE_CURVE('',#993,#994,#196,.T.);
#1281=EDGE_CURVE('',#995,#996,#197,.T.);
#1282=EDGE_CURVE('',#996,#997,#578,.T.);
#1283=EDGE_CURVE('',#997,#997,#198,.T.);
#1284=EDGE_CURVE('',#996,#998,#199,.T.);
#1285=EDGE_CURVE('',#998,#999,#579,.T.);
#1286=EDGE_CURVE('',#883,#999,#200,.T.);
#1287=EDGE_CURVE('',#891,#890,#201,.T.);
#1288=EDGE_CURVE('',#899,#898,#202,.T.);
#1289=EDGE_CURVE('',#907,#906,#203,.T.);
#1290=EDGE_CURVE('',#915,#914,#204,.T.);
#1291=EDGE_CURVE('',#923,#922,#205,.T.);
#1292=EDGE_CURVE('',#931,#930,#206,.T.);
#1293=EDGE_CURVE('',#939,#938,#207,.T.);
#1294=EDGE_CURVE('',#947,#946,#208,.T.);
#1295=EDGE_CURVE('',#955,#954,#209,.T.);
#1296=EDGE_CURVE('',#963,#962,#210,.T.);
#1297=EDGE_CURVE('',#971,#970,#211,.T.);
#1298=EDGE_CURVE('',#979,#978,#212,.T.);
#1299=EDGE_CURVE('',#987,#986,#213,.T.);
#1300=EDGE_CURVE('',#1000,#994,#214,.T.);
#1301=EDGE_CURVE('',#1000,#995,#580,.T.);
#1302=EDGE_CURVE('',#1000,#1001,#215,.T.);
#1303=EDGE_CURVE('',#1001,#1002,#581,.T.);
#1304=EDGE_CURVE('',#1002,#995,#216,.T.);
#1305=EDGE_CURVE('',#1003,#1002,#217,.T.);
#1306=EDGE_CURVE('',#998,#1003,#218,.T.);
#1307=EDGE_CURVE('',#1004,#1001,#219,.T.);
#1308=EDGE_CURVE('',#1004,#1003,#582,.T.);
#1309=EDGE_CURVE('',#1004,#999,#220,.T.);
#1310=EDGE_CURVE('',#1005,#1005,#221,.T.);
#1311=EDGE_CURVE('',#1006,#1006,#222,.T.);
#1312=EDGE_CURVE('',#1007,#1007,#223,.T.);
#1313=EDGE_CURVE('',#1007,#1006,#583,.T.);
#1314=EDGE_CURVE('',#1008,#1008,#224,.T.);
#1315=EDGE_CURVE('',#1008,#881,#584,.T.);
#1316=EDGE_CURVE('',#882,#1007,#585,.T.);
#1317=EDGE_CURVE('',#1008,#1009,#586,.T.);
#1318=EDGE_CURVE('',#1009,#1009,#225,.T.);
#1319=EDGE_CURVE('',#1010,#1010,#226,.T.);
#1320=EDGE_CURVE('',#1011,#1011,#227,.T.);
#1321=EDGE_CURVE('',#1011,#1010,#587,.T.);
#1322=EDGE_CURVE('',#1011,#1012,#588,.T.);
#1323=EDGE_CURVE('',#1012,#1012,#228,.T.);
#1324=EDGE_CURVE('',#1013,#1013,#229,.T.);
#1325=EDGE_CURVE('',#879,#1013,#589,.T.);
#1326=EDGE_CURVE('',#875,#1014,#590,.T.);
#1327=EDGE_CURVE('',#1014,#1014,#230,.T.);
#1328=EDGE_CURVE('',#1015,#1015,#231,.T.);
#1329=EDGE_CURVE('',#1016,#1016,#232,.T.);
#1330=EDGE_CURVE('',#1016,#1015,#591,.T.);
#1331=EDGE_CURVE('',#1016,#1017,#592,.T.);
#1332=EDGE_CURVE('',#1017,#1017,#233,.T.);
#1333=EDGE_CURVE('',#1018,#1018,#234,.T.);
#1334=EDGE_CURVE('',#1019,#1019,#235,.T.);
#1335=EDGE_CURVE('',#1019,#1018,#593,.T.);
#1336=EDGE_CURVE('',#1020,#1020,#236,.T.);
#1337=EDGE_CURVE('',#1020,#1019,#594,.T.);
#1338=EDGE_CURVE('',#1020,#1005,#595,.T.);
#1471=ORIENTED_EDGE('',*,*,#1109,.F.);
#1472=ORIENTED_EDGE('',*,*,#1110,.F.);
#1473=ORIENTED_EDGE('',*,*,#1111,.F.);
#1474=ORIENTED_EDGE('',*,*,#1112,.T.);
#1475=ORIENTED_EDGE('',*,*,#1113,.F.);
#1476=ORIENTED_EDGE('',*,*,#1114,.F.);
#1477=ORIENTED_EDGE('',*,*,#1112,.F.);
#1478=ORIENTED_EDGE('',*,*,#1115,.F.);
#1479=ORIENTED_EDGE('',*,*,#1116,.T.);
#1480=ORIENTED_EDGE('',*,*,#1117,.T.);
#1481=ORIENTED_EDGE('',*,*,#1118,.T.);
#1482=ORIENTED_EDGE('',*,*,#1119,.T.);
#1483=ORIENTED_EDGE('',*,*,#1120,.T.);
#1484=ORIENTED_EDGE('',*,*,#1119,.F.);
#1485=ORIENTED_EDGE('',*,*,#1121,.T.);
#1486=ORIENTED_EDGE('',*,*,#1109,.T.);
#1487=ORIENTED_EDGE('',*,*,#1111,.T.);
#1488=ORIENTED_EDGE('',*,*,#1122,.T.);
#1489=ORIENTED_EDGE('',*,*,#1116,.F.);
#1490=ORIENTED_EDGE('',*,*,#1122,.F.);
#1491=ORIENTED_EDGE('',*,*,#1110,.T.);
#1492=ORIENTED_EDGE('',*,*,#1121,.F.);
#1493=ORIENTED_EDGE('',*,*,#1118,.F.);
#1494=ORIENTED_EDGE('',*,*,#1123,.T.);
#1495=ORIENTED_EDGE('',*,*,#1124,.F.);
#1496=ORIENTED_EDGE('',*,*,#1125,.F.);
#1497=ORIENTED_EDGE('',*,*,#1126,.F.);
#1498=ORIENTED_EDGE('',*,*,#1123,.F.);
#1499=ORIENTED_EDGE('',*,*,#1117,.F.);
#1500=ORIENTED_EDGE('',*,*,#1127,.F.);
#1501=ORIENTED_EDGE('',*,*,#1128,.T.);
#1502=ORIENTED_EDGE('',*,*,#1129,.T.);
#1503=ORIENTED_EDGE('',*,*,#1130,.T.);
#1504=ORIENTED_EDGE('',*,*,#1131,.F.);
#1505=ORIENTED_EDGE('',*,*,#1130,.F.);
#1506=ORIENTED_EDGE('',*,*,#1132,.F.);
#1507=ORIENTED_EDGE('',*,*,#1133,.F.);
#1508=ORIENTED_EDGE('',*,*,#1134,.F.);
#1509=ORIENTED_EDGE('',*,*,#1135,.T.);
#1510=ORIENTED_EDGE('',*,*,#1132,.T.);
#1511=ORIENTED_EDGE('',*,*,#1129,.F.);
#1512=ORIENTED_EDGE('',*,*,#1136,.F.);
#1513=ORIENTED_EDGE('',*,*,#1133,.T.);
#1514=ORIENTED_EDGE('',*,*,#1135,.F.);
#1515=ORIENTED_EDGE('',*,*,#1137,.T.);
#1516=ORIENTED_EDGE('',*,*,#1138,.F.);
#1517=ORIENTED_EDGE('',*,*,#1139,.T.);
#1518=ORIENTED_EDGE('',*,*,#1140,.T.);
#1519=ORIENTED_EDGE('',*,*,#1141,.T.);
#1520=ORIENTED_EDGE('',*,*,#1142,.F.);
#1521=ORIENTED_EDGE('',*,*,#1141,.F.);
#1522=ORIENTED_EDGE('',*,*,#1143,.F.);
#1523=ORIENTED_EDGE('',*,*,#1144,.F.);
#1524=ORIENTED_EDGE('',*,*,#1145,.F.);
#1525=ORIENTED_EDGE('',*,*,#1146,.T.);
#1526=ORIENTED_EDGE('',*,*,#1143,.T.);
#1527=ORIENTED_EDGE('',*,*,#1140,.F.);
#1528=ORIENTED_EDGE('',*,*,#1147,.F.);
#1529=ORIENTED_EDGE('',*,*,#1144,.T.);
#1530=ORIENTED_EDGE('',*,*,#1146,.F.);
#1531=ORIENTED_EDGE('',*,*,#1148,.T.);
#1532=ORIENTED_EDGE('',*,*,#1149,.F.);
#1533=ORIENTED_EDGE('',*,*,#1150,.T.);
#1534=ORIENTED_EDGE('',*,*,#1151,.T.);
#1535=ORIENTED_EDGE('',*,*,#1152,.T.);
#1536=ORIENTED_EDGE('',*,*,#1153,.F.);
#1537=ORIENTED_EDGE('',*,*,#1152,.F.);
#1538=ORIENTED_EDGE('',*,*,#1154,.F.);
#1539=ORIENTED_EDGE('',*,*,#1155,.F.);
#1540=ORIENTED_EDGE('',*,*,#1156,.F.);
#1541=ORIENTED_EDGE('',*,*,#1157,.T.);
#1542=ORIENTED_EDGE('',*,*,#1154,.T.);
#1543=ORIENTED_EDGE('',*,*,#1151,.F.);
#1544=ORIENTED_EDGE('',*,*,#1158,.F.);
#1545=ORIENTED_EDGE('',*,*,#1155,.T.);
#1546=ORIENTED_EDGE('',*,*,#1157,.F.);
#1547=ORIENTED_EDGE('',*,*,#1159,.T.);
#1548=ORIENTED_EDGE('',*,*,#1160,.F.);
#1549=ORIENTED_EDGE('',*,*,#1161,.T.);
#1550=ORIENTED_EDGE('',*,*,#1162,.T.);
#1551=ORIENTED_EDGE('',*,*,#1163,.T.);
#1552=ORIENTED_EDGE('',*,*,#1164,.F.);
#1553=ORIENTED_EDGE('',*,*,#1163,.F.);
#1554=ORIENTED_EDGE('',*,*,#1165,.F.);
#1555=ORIENTED_EDGE('',*,*,#1166,.F.);
#1556=ORIENTED_EDGE('',*,*,#1167,.F.);
#1557=ORIENTED_EDGE('',*,*,#1168,.T.);
#1558=ORIENTED_EDGE('',*,*,#1165,.T.);
#1559=ORIENTED_EDGE('',*,*,#1162,.F.);
#1560=ORIENTED_EDGE('',*,*,#1169,.F.);
#1561=ORIENTED_EDGE('',*,*,#1166,.T.);
#1562=ORIENTED_EDGE('',*,*,#1168,.F.);
#1563=ORIENTED_EDGE('',*,*,#1170,.T.);
#1564=ORIENTED_EDGE('',*,*,#1171,.F.);
#1565=ORIENTED_EDGE('',*,*,#1172,.T.);
#1566=ORIENTED_EDGE('',*,*,#1173,.T.);
#1567=ORIENTED_EDGE('',*,*,#1174,.T.);
#1568=ORIENTED_EDGE('',*,*,#1175,.F.);
#1569=ORIENTED_EDGE('',*,*,#1174,.F.);
#1570=ORIENTED_EDGE('',*,*,#1176,.F.);
#1571=ORIENTED_EDGE('',*,*,#1177,.F.);
#1572=ORIENTED_EDGE('',*,*,#1178,.F.);
#1573=ORIENTED_EDGE('',*,*,#1179,.T.);
#1574=ORIENTED_EDGE('',*,*,#1176,.T.);
#1575=ORIENTED_EDGE('',*,*,#1173,.F.);
#1576=ORIENTED_EDGE('',*,*,#1180,.F.);
#1577=ORIENTED_EDGE('',*,*,#1177,.T.);
#1578=ORIENTED_EDGE('',*,*,#1179,.F.);
#1579=ORIENTED_EDGE('',*,*,#1181,.T.);
#1580=ORIENTED_EDGE('',*,*,#1182,.F.);
#1581=ORIENTED_EDGE('',*,*,#1183,.T.);
#1582=ORIENTED_EDGE('',*,*,#1184,.T.);
#1583=ORIENTED_EDGE('',*,*,#1185,.T.);
#1584=ORIENTED_EDGE('',*,*,#1186,.F.);
#1585=ORIENTED_EDGE('',*,*,#1185,.F.);
#1586=ORIENTED_EDGE('',*,*,#1187,.F.);
#1587=ORIENTED_EDGE('',*,*,#1188,.F.);
#1588=ORIENTED_EDGE('',*,*,#1189,.F.);
#1589=ORIENTED_EDGE('',*,*,#1190,.T.);
#1590=ORIENTED_EDGE('',*,*,#1187,.T.);
#1591=ORIENTED_EDGE('',*,*,#1184,.F.);
#1592=ORIENTED_EDGE('',*,*,#1191,.F.);
#1593=ORIENTED_EDGE('',*,*,#1188,.T.);
#1594=ORIENTED_EDGE('',*,*,#1190,.F.);
#1595=ORIENTED_EDGE('',*,*,#1192,.T.);
#1596=ORIENTED_EDGE('',*,*,#1193,.F.);
#1597=ORIENTED_EDGE('',*,*,#1194,.T.);
#1598=ORIENTED_EDGE('',*,*,#1195,.T.);
#1599=ORIENTED_EDGE('',*,*,#1196,.T.);
#1600=ORIENTED_EDGE('',*,*,#1197,.F.);
#1601=ORIENTED_EDGE('',*,*,#1196,.F.);
#1602=ORIENTED_EDGE('',*,*,#1198,.F.);
#1603=ORIENTED_EDGE('',*,*,#1199,.F.);
#1604=ORIENTED_EDGE('',*,*,#1200,.F.);
#1605=ORIENTED_EDGE('',*,*,#1201,.T.);
#1606=ORIENTED_EDGE('',*,*,#1198,.T.);
#1607=ORIENTED_EDGE('',*,*,#1195,.F.);
#1608=ORIENTED_EDGE('',*,*,#1202,.F.);
#1609=ORIENTED_EDGE('',*,*,#1199,.T.);
#1610=ORIENTED_EDGE('',*,*,#1201,.F.);
#1611=ORIENTED_EDGE('',*,*,#1203,.T.);
#1612=ORIENTED_EDGE('',*,*,#1204,.F.);
#1613=ORIENTED_EDGE('',*,*,#1205,.T.);
#1614=ORIENTED_EDGE('',*,*,#1206,.T.);
#1615=ORIENTED_EDGE('',*,*,#1207,.T.);
#1616=ORIENTED_EDGE('',*,*,#1208,.F.);
#1617=ORIENTED_EDGE('',*,*,#1207,.F.);
#1618=ORIENTED_EDGE('',*,*,#1209,.F.);
#1619=ORIENTED_EDGE('',*,*,#1210,.F.);
#1620=ORIENTED_EDGE('',*,*,#1211,.F.);
#1621=ORIENTED_EDGE('',*,*,#1212,.T.);
#1622=ORIENTED_EDGE('',*,*,#1209,.T.);
#1623=ORIENTED_EDGE('',*,*,#1206,.F.);
#1624=ORIENTED_EDGE('',*,*,#1213,.F.);
#1625=ORIENTED_EDGE('',*,*,#1210,.T.);
#1626=ORIENTED_EDGE('',*,*,#1212,.F.);
#1627=ORIENTED_EDGE('',*,*,#1214,.T.);
#1628=ORIENTED_EDGE('',*,*,#1215,.F.);
#1629=ORIENTED_EDGE('',*,*,#1216,.T.);
#1630=ORIENTED_EDGE('',*,*,#1217,.T.);
#1631=ORIENTED_EDGE('',*,*,#1218,.T.);
#1632=ORIENTED_EDGE('',*,*,#1219,.F.);
#1633=ORIENTED_EDGE('',*,*,#1218,.F.);
#1634=ORIENTED_EDGE('',*,*,#1220,.F.);
#1635=ORIENTED_EDGE('',*,*,#1221,.F.);
#1636=ORIENTED_EDGE('',*,*,#1222,.F.);
#1637=ORIENTED_EDGE('',*,*,#1223,.T.);
#1638=ORIENTED_EDGE('',*,*,#1220,.T.);
#1639=ORIENTED_EDGE('',*,*,#1217,.F.);
#1640=ORIENTED_EDGE('',*,*,#1224,.F.);
#1641=ORIENTED_EDGE('',*,*,#1221,.T.);
#1642=ORIENTED_EDGE('',*,*,#1223,.F.);
#1643=ORIENTED_EDGE('',*,*,#1225,.T.);
#1644=ORIENTED_EDGE('',*,*,#1226,.F.);
#1645=ORIENTED_EDGE('',*,*,#1227,.T.);
#1646=ORIENTED_EDGE('',*,*,#1228,.T.);
#1647=ORIENTED_EDGE('',*,*,#1229,.T.);
#1648=ORIENTED_EDGE('',*,*,#1230,.F.);
#1649=ORIENTED_EDGE('',*,*,#1229,.F.);
#1650=ORIENTED_EDGE('',*,*,#1231,.F.);
#1651=ORIENTED_EDGE('',*,*,#1232,.F.);
#1652=ORIENTED_EDGE('',*,*,#1233,.F.);
#1653=ORIENTED_EDGE('',*,*,#1234,.T.);
#1654=ORIENTED_EDGE('',*,*,#1231,.T.);
#1655=ORIENTED_EDGE('',*,*,#1228,.F.);
#1656=ORIENTED_EDGE('',*,*,#1235,.F.);
#1657=ORIENTED_EDGE('',*,*,#1232,.T.);
#1658=ORIENTED_EDGE('',*,*,#1234,.F.);
#1659=ORIENTED_EDGE('',*,*,#1236,.T.);
#1660=ORIENTED_EDGE('',*,*,#1237,.F.);
#1661=ORIENTED_EDGE('',*,*,#1238,.T.);
#1662=ORIENTED_EDGE('',*,*,#1239,.T.);
#1663=ORIENTED_EDGE('',*,*,#1240,.T.);
#1664=ORIENTED_EDGE('',*,*,#1241,.F.);
#1665=ORIENTED_EDGE('',*,*,#1240,.F.);
#1666=ORIENTED_EDGE('',*,*,#1242,.F.);
#1667=ORIENTED_EDGE('',*,*,#1243,.F.);
#1668=ORIENTED_EDGE('',*,*,#1244,.F.);
#1669=ORIENTED_EDGE('',*,*,#1245,.T.);
#1670=ORIENTED_EDGE('',*,*,#1242,.T.);
#1671=ORIENTED_EDGE('',*,*,#1239,.F.);
#1672=ORIENTED_EDGE('',*,*,#1246,.F.);
#1673=ORIENTED_EDGE('',*,*,#1243,.T.);
#1674=ORIENTED_EDGE('',*,*,#1245,.F.);
#1675=ORIENTED_EDGE('',*,*,#1247,.T.);
#1676=ORIENTED_EDGE('',*,*,#1248,.F.);
#1677=ORIENTED_EDGE('',*,*,#1249,.T.);
#1678=ORIENTED_EDGE('',*,*,#1250,.T.);
#1679=ORIENTED_EDGE('',*,*,#1251,.T.);
#1680=ORIENTED_EDGE('',*,*,#1252,.F.);
#1681=ORIENTED_EDGE('',*,*,#1251,.F.);
#1682=ORIENTED_EDGE('',*,*,#1253,.F.);
#1683=ORIENTED_EDGE('',*,*,#1254,.F.);
#1684=ORIENTED_EDGE('',*,*,#1255,.F.);
#1685=ORIENTED_EDGE('',*,*,#1256,.T.);
#1686=ORIENTED_EDGE('',*,*,#1253,.T.);
#1687=ORIENTED_EDGE('',*,*,#1250,.F.);
#1688=ORIENTED_EDGE('',*,*,#1257,.F.);
#1689=ORIENTED_EDGE('',*,*,#1254,.T.);
#1690=ORIENTED_EDGE('',*,*,#1256,.F.);
#1691=ORIENTED_EDGE('',*,*,#1258,.T.);
#1692=ORIENTED_EDGE('',*,*,#1259,.F.);
#1693=ORIENTED_EDGE('',*,*,#1260,.T.);
#1694=ORIENTED_EDGE('',*,*,#1261,.T.);
#1695=ORIENTED_EDGE('',*,*,#1262,.T.);
#1696=ORIENTED_EDGE('',*,*,#1263,.F.);
#1697=ORIENTED_EDGE('',*,*,#1262,.F.);
#1698=ORIENTED_EDGE('',*,*,#1264,.F.);
#1699=ORIENTED_EDGE('',*,*,#1265,.F.);
#1700=ORIENTED_EDGE('',*,*,#1266,.F.);
#1701=ORIENTED_EDGE('',*,*,#1267,.T.);
#1702=ORIENTED_EDGE('',*,*,#1264,.T.);
#1703=ORIENTED_EDGE('',*,*,#1261,.F.);
#1704=ORIENTED_EDGE('',*,*,#1268,.F.);
#1705=ORIENTED_EDGE('',*,*,#1265,.T.);
#1706=ORIENTED_EDGE('',*,*,#1267,.F.);
#1707=ORIENTED_EDGE('',*,*,#1269,.T.);
#1708=ORIENTED_EDGE('',*,*,#1270,.F.);
#1709=ORIENTED_EDGE('',*,*,#1271,.T.);
#1710=ORIENTED_EDGE('',*,*,#1272,.T.);
#1711=ORIENTED_EDGE('',*,*,#1273,.T.);
#1712=ORIENTED_EDGE('',*,*,#1274,.F.);
#1713=ORIENTED_EDGE('',*,*,#1273,.F.);
#1714=ORIENTED_EDGE('',*,*,#1275,.F.);
#1715=ORIENTED_EDGE('',*,*,#1276,.F.);
#1716=ORIENTED_EDGE('',*,*,#1277,.F.);
#1717=ORIENTED_EDGE('',*,*,#1278,.T.);
#1718=ORIENTED_EDGE('',*,*,#1275,.T.);
#1719=ORIENTED_EDGE('',*,*,#1272,.F.);
#1720=ORIENTED_EDGE('',*,*,#1279,.F.);
#1721=ORIENTED_EDGE('',*,*,#1276,.T.);
#1722=ORIENTED_EDGE('',*,*,#1278,.F.);
#1723=ORIENTED_EDGE('',*,*,#1280,.T.);
#1724=ORIENTED_EDGE('',*,*,#1281,.T.);
#1725=ORIENTED_EDGE('',*,*,#1282,.T.);
#1726=ORIENTED_EDGE('',*,*,#1283,.T.);
#1727=ORIENTED_EDGE('',*,*,#1282,.F.);
#1728=ORIENTED_EDGE('',*,*,#1284,.T.);
#1729=ORIENTED_EDGE('',*,*,#1285,.T.);
#1730=ORIENTED_EDGE('',*,*,#1286,.F.);
#1731=ORIENTED_EDGE('',*,*,#1127,.T.);
#1732=ORIENTED_EDGE('',*,*,#1131,.T.);
#1733=ORIENTED_EDGE('',*,*,#1136,.T.);
#1734=ORIENTED_EDGE('',*,*,#1287,.F.);
#1735=ORIENTED_EDGE('',*,*,#1138,.T.);
#1736=ORIENTED_EDGE('',*,*,#1142,.T.);
#1737=ORIENTED_EDGE('',*,*,#1147,.T.);
#1738=ORIENTED_EDGE('',*,*,#1288,.F.);
#1739=ORIENTED_EDGE('',*,*,#1149,.T.);
#1740=ORIENTED_EDGE('',*,*,#1153,.T.);
#1741=ORIENTED_EDGE('',*,*,#1158,.T.);
#1742=ORIENTED_EDGE('',*,*,#1289,.F.);
#1743=ORIENTED_EDGE('',*,*,#1160,.T.);
#1744=ORIENTED_EDGE('',*,*,#1164,.T.);
#1745=ORIENTED_EDGE('',*,*,#1169,.T.);
#1746=ORIENTED_EDGE('',*,*,#1290,.F.);
#1747=ORIENTED_EDGE('',*,*,#1171,.T.);
#1748=ORIENTED_EDGE('',*,*,#1175,.T.);
#1749=ORIENTED_EDGE('',*,*,#1180,.T.);
#1750=ORIENTED_EDGE('',*,*,#1291,.F.);
#1751=ORIENTED_EDGE('',*,*,#1182,.T.);
#1752=ORIENTED_EDGE('',*,*,#1186,.T.);
#1753=ORIENTED_EDGE('',*,*,#1191,.T.);
#1754=ORIENTED_EDGE('',*,*,#1292,.F.);
#1755=ORIENTED_EDGE('',*,*,#1193,.T.);
#1756=ORIENTED_EDGE('',*,*,#1197,.T.);
#1757=ORIENTED_EDGE('',*,*,#1202,.T.);
#1758=ORIENTED_EDGE('',*,*,#1293,.F.);
#1759=ORIENTED_EDGE('',*,*,#1204,.T.);
#1760=ORIENTED_EDGE('',*,*,#1208,.T.);
#1761=ORIENTED_EDGE('',*,*,#1213,.T.);
#1762=ORIENTED_EDGE('',*,*,#1294,.F.);
#1763=ORIENTED_EDGE('',*,*,#1215,.T.);
#1764=ORIENTED_EDGE('',*,*,#1219,.T.);
#1765=ORIENTED_EDGE('',*,*,#1224,.T.);
#1766=ORIENTED_EDGE('',*,*,#1295,.F.);
#1767=ORIENTED_EDGE('',*,*,#1226,.T.);
#1768=ORIENTED_EDGE('',*,*,#1230,.T.);
#1769=ORIENTED_EDGE('',*,*,#1235,.T.);
#1770=ORIENTED_EDGE('',*,*,#1296,.F.);
#1771=ORIENTED_EDGE('',*,*,#1237,.T.);
#1772=ORIENTED_EDGE('',*,*,#1241,.T.);
#1773=ORIENTED_EDGE('',*,*,#1246,.T.);
#1774=ORIENTED_EDGE('',*,*,#1297,.F.);
#1775=ORIENTED_EDGE('',*,*,#1248,.T.);
#1776=ORIENTED_EDGE('',*,*,#1252,.T.);
#1777=ORIENTED_EDGE('',*,*,#1257,.T.);
#1778=ORIENTED_EDGE('',*,*,#1298,.F.);
#1779=ORIENTED_EDGE('',*,*,#1259,.T.);
#1780=ORIENTED_EDGE('',*,*,#1263,.T.);
#1781=ORIENTED_EDGE('',*,*,#1268,.T.);
#1782=ORIENTED_EDGE('',*,*,#1299,.F.);
#1783=ORIENTED_EDGE('',*,*,#1270,.T.);
#1784=ORIENTED_EDGE('',*,*,#1274,.T.);
#1785=ORIENTED_EDGE('',*,*,#1279,.T.);
#1786=ORIENTED_EDGE('',*,*,#1300,.F.);
#1787=ORIENTED_EDGE('',*,*,#1301,.T.);
#1788=ORIENTED_EDGE('',*,*,#1301,.F.);
#1789=ORIENTED_EDGE('',*,*,#1302,.T.);
#1790=ORIENTED_EDGE('',*,*,#1303,.T.);
#1791=ORIENTED_EDGE('',*,*,#1304,.T.);
#1792=ORIENTED_EDGE('',*,*,#1281,.F.);
#1793=ORIENTED_EDGE('',*,*,#1304,.F.);
#1794=ORIENTED_EDGE('',*,*,#1305,.F.);
#1795=ORIENTED_EDGE('',*,*,#1306,.F.);
#1796=ORIENTED_EDGE('',*,*,#1284,.F.);
#1797=ORIENTED_EDGE('',*,*,#1307,.F.);
#1798=ORIENTED_EDGE('',*,*,#1308,.T.);
#1799=ORIENTED_EDGE('',*,*,#1305,.T.);
#1800=ORIENTED_EDGE('',*,*,#1303,.F.);
#1801=ORIENTED_EDGE('',*,*,#1285,.F.);
#1802=ORIENTED_EDGE('',*,*,#1306,.T.);
#1803=ORIENTED_EDGE('',*,*,#1308,.F.);
#1804=ORIENTED_EDGE('',*,*,#1309,.T.);
#1805=ORIENTED_EDGE('',*,*,#1310,.T.);
#1806=ORIENTED_EDGE('',*,*,#1283,.F.);
#1807=ORIENTED_EDGE('',*,*,#1311,.F.);
#1808=ORIENTED_EDGE('',*,*,#1286,.T.);
#1809=ORIENTED_EDGE('',*,*,#1309,.F.);
#1810=ORIENTED_EDGE('',*,*,#1307,.T.);
#1811=ORIENTED_EDGE('',*,*,#1302,.F.);
#1812=ORIENTED_EDGE('',*,*,#1300,.T.);
#1813=ORIENTED_EDGE('',*,*,#1280,.F.);
#1814=ORIENTED_EDGE('',*,*,#1277,.T.);
#1815=ORIENTED_EDGE('',*,*,#1271,.F.);
#1816=ORIENTED_EDGE('',*,*,#1299,.T.);
#1817=ORIENTED_EDGE('',*,*,#1269,.F.);
#1818=ORIENTED_EDGE('',*,*,#1266,.T.);
#1819=ORIENTED_EDGE('',*,*,#1260,.F.);
#1820=ORIENTED_EDGE('',*,*,#1298,.T.);
#1821=ORIENTED_EDGE('',*,*,#1258,.F.);
#1822=ORIENTED_EDGE('',*,*,#1255,.T.);
#1823=ORIENTED_EDGE('',*,*,#1249,.F.);
#1824=ORIENTED_EDGE('',*,*,#1297,.T.);
#1825=ORIENTED_EDGE('',*,*,#1247,.F.);
#1826=ORIENTED_EDGE('',*,*,#1244,.T.);
#1827=ORIENTED_EDGE('',*,*,#1238,.F.);
#1828=ORIENTED_EDGE('',*,*,#1296,.T.);
#1829=ORIENTED_EDGE('',*,*,#1236,.F.);
#1830=ORIENTED_EDGE('',*,*,#1233,.T.);
#1831=ORIENTED_EDGE('',*,*,#1227,.F.);
#1832=ORIENTED_EDGE('',*,*,#1295,.T.);
#1833=ORIENTED_EDGE('',*,*,#1225,.F.);
#1834=ORIENTED_EDGE('',*,*,#1222,.T.);
#1835=ORIENTED_EDGE('',*,*,#1216,.F.);
#1836=ORIENTED_EDGE('',*,*,#1294,.T.);
#1837=ORIENTED_EDGE('',*,*,#1214,.F.);
#1838=ORIENTED_EDGE('',*,*,#1211,.T.);
#1839=ORIENTED_EDGE('',*,*,#1205,.F.);
#1840=ORIENTED_EDGE('',*,*,#1293,.T.);
#1841=ORIENTED_EDGE('',*,*,#1203,.F.);
#1842=ORIENTED_EDGE('',*,*,#1200,.T.);
#1843=ORIENTED_EDGE('',*,*,#1194,.F.);
#1844=ORIENTED_EDGE('',*,*,#1292,.T.);
#1845=ORIENTED_EDGE('',*,*,#1192,.F.);
#1846=ORIENTED_EDGE('',*,*,#1189,.T.);
#1847=ORIENTED_EDGE('',*,*,#1183,.F.);
#1848=ORIENTED_EDGE('',*,*,#1291,.T.);
#1849=ORIENTED_EDGE('',*,*,#1181,.F.);
#1850=ORIENTED_EDGE('',*,*,#1178,.T.);
#1851=ORIENTED_EDGE('',*,*,#1172,.F.);
#1852=ORIENTED_EDGE('',*,*,#1290,.T.);
#1853=ORIENTED_EDGE('',*,*,#1170,.F.);
#1854=ORIENTED_EDGE('',*,*,#1167,.T.);
#1855=ORIENTED_EDGE('',*,*,#1161,.F.);
#1856=ORIENTED_EDGE('',*,*,#1289,.T.);
#1857=ORIENTED_EDGE('',*,*,#1159,.F.);
#1858=ORIENTED_EDGE('',*,*,#1156,.T.);
#1859=ORIENTED_EDGE('',*,*,#1150,.F.);
#1860=ORIENTED_EDGE('',*,*,#1288,.T.);
#1861=ORIENTED_EDGE('',*,*,#1148,.F.);
#1862=ORIENTED_EDGE('',*,*,#1145,.T.);
#1863=ORIENTED_EDGE('',*,*,#1139,.F.);
#1864=ORIENTED_EDGE('',*,*,#1287,.T.);
#1865=ORIENTED_EDGE('',*,*,#1137,.F.);
#1866=ORIENTED_EDGE('',*,*,#1134,.T.);
#1867=ORIENTED_EDGE('',*,*,#1128,.F.);
#1868=ORIENTED_EDGE('',*,*,#1312,.F.);
#1869=ORIENTED_EDGE('',*,*,#1313,.T.);
#1870=ORIENTED_EDGE('',*,*,#1311,.T.);
#1871=ORIENTED_EDGE('',*,*,#1313,.F.);
#1872=ORIENTED_EDGE('',*,*,#1314,.F.);
#1873=ORIENTED_EDGE('',*,*,#1315,.T.);
#1874=ORIENTED_EDGE('',*,*,#1124,.T.);
#1875=ORIENTED_EDGE('',*,*,#1126,.T.);
#1876=ORIENTED_EDGE('',*,*,#1316,.T.);
#1877=ORIENTED_EDGE('',*,*,#1312,.T.);
#1878=ORIENTED_EDGE('',*,*,#1316,.F.);
#1879=ORIENTED_EDGE('',*,*,#1125,.T.);
#1880=ORIENTED_EDGE('',*,*,#1315,.F.);
#1881=ORIENTED_EDGE('',*,*,#1113,.T.);
#1882=ORIENTED_EDGE('',*,*,#1114,.T.);
#1883=ORIENTED_EDGE('',*,*,#1314,.T.);
#1884=ORIENTED_EDGE('',*,*,#1317,.T.);
#1885=ORIENTED_EDGE('',*,*,#1318,.F.);
#1886=ORIENTED_EDGE('',*,*,#1317,.F.);
#1887=ORIENTED_EDGE('',*,*,#1318,.T.);
#1888=ORIENTED_EDGE('',*,*,#1319,.F.);
#1889=ORIENTED_EDGE('',*,*,#1320,.F.);
#1890=ORIENTED_EDGE('',*,*,#1321,.T.);
#1891=ORIENTED_EDGE('',*,*,#1319,.T.);
#1892=ORIENTED_EDGE('',*,*,#1321,.F.);
#1893=ORIENTED_EDGE('',*,*,#1320,.T.);
#1894=ORIENTED_EDGE('',*,*,#1322,.T.);
#1895=ORIENTED_EDGE('',*,*,#1323,.F.);
#1896=ORIENTED_EDGE('',*,*,#1322,.F.);
#1897=ORIENTED_EDGE('',*,*,#1323,.T.);
#1898=ORIENTED_EDGE('',*,*,#1324,.F.);
#1899=ORIENTED_EDGE('',*,*,#1120,.F.);
#1900=ORIENTED_EDGE('',*,*,#1325,.T.);
#1901=ORIENTED_EDGE('',*,*,#1324,.T.);
#1902=ORIENTED_EDGE('',*,*,#1325,.F.);
#1903=ORIENTED_EDGE('',*,*,#1115,.T.);
#1904=ORIENTED_EDGE('',*,*,#1326,.T.);
#1905=ORIENTED_EDGE('',*,*,#1327,.F.);
#1906=ORIENTED_EDGE('',*,*,#1326,.F.);
#1907=ORIENTED_EDGE('',*,*,#1328,.F.);
#1908=ORIENTED_EDGE('',*,*,#1327,.T.);
#1909=ORIENTED_EDGE('',*,*,#1329,.F.);
#1910=ORIENTED_EDGE('',*,*,#1330,.T.);
#1911=ORIENTED_EDGE('',*,*,#1328,.T.);
#1912=ORIENTED_EDGE('',*,*,#1330,.F.);
#1913=ORIENTED_EDGE('',*,*,#1329,.T.);
#1914=ORIENTED_EDGE('',*,*,#1331,.T.);
#1915=ORIENTED_EDGE('',*,*,#1332,.F.);
#1916=ORIENTED_EDGE('',*,*,#1331,.F.);
#1917=ORIENTED_EDGE('',*,*,#1333,.F.);
#1918=ORIENTED_EDGE('',*,*,#1332,.T.);
#1919=ORIENTED_EDGE('',*,*,#1334,.F.);
#1920=ORIENTED_EDGE('',*,*,#1335,.T.);
#1921=ORIENTED_EDGE('',*,*,#1333,.T.);
#1922=ORIENTED_EDGE('',*,*,#1335,.F.);
#1923=ORIENTED_EDGE('',*,*,#1336,.F.);
#1924=ORIENTED_EDGE('',*,*,#1337,.T.);
#1925=ORIENTED_EDGE('',*,*,#1334,.T.);
#1926=ORIENTED_EDGE('',*,*,#1337,.F.);
#1927=ORIENTED_EDGE('',*,*,#1336,.T.);
#1928=ORIENTED_EDGE('',*,*,#1338,.T.);
#1929=ORIENTED_EDGE('',*,*,#1310,.F.);
#1930=ORIENTED_EDGE('',*,*,#1338,.F.);
#2195=CYLINDRICAL_SURFACE('',#2445,2.00054127207588);
#2196=CYLINDRICAL_SURFACE('',#2446,2.50080065552765);
#2197=CYLINDRICAL_SURFACE('',#2449,2.00007126058529);
#2198=CYLINDRICAL_SURFACE('',#2450,0.124032861755453);
#2199=CYLINDRICAL_SURFACE('',#2457,0.749041401963156);
#2200=CYLINDRICAL_SURFACE('',#2459,0.124032861755453);
#2201=CYLINDRICAL_SURFACE('',#2461,0.124032861755453);
#2202=CYLINDRICAL_SURFACE('',#2468,0.749041401963156);
#2203=CYLINDRICAL_SURFACE('',#2470,0.124032861755453);
#2204=CYLINDRICAL_SURFACE('',#2472,0.124032861755453);
#2205=CYLINDRICAL_SURFACE('',#2479,0.749041401963155);
#2206=CYLINDRICAL_SURFACE('',#2481,0.124032861755453);
#2207=CYLINDRICAL_SURFACE('',#2483,0.124032861755453);
#2208=CYLINDRICAL_SURFACE('',#2490,0.749041401963156);
#2209=CYLINDRICAL_SURFACE('',#2492,0.124032861755453);
#2210=CYLINDRICAL_SURFACE('',#2494,0.124032861755453);
#2211=CYLINDRICAL_SURFACE('',#2501,0.749041401963155);
#2212=CYLINDRICAL_SURFACE('',#2503,0.124032861755453);
#2213=CYLINDRICAL_SURFACE('',#2505,0.124032861755453);
#2214=CYLINDRICAL_SURFACE('',#2512,0.749041401963156);
#2215=CYLINDRICAL_SURFACE('',#2514,0.124032861755453);
#2216=CYLINDRICAL_SURFACE('',#2516,0.124032861755453);
#2217=CYLINDRICAL_SURFACE('',#2523,0.749041401963155);
#2218=CYLINDRICAL_SURFACE('',#2525,0.124032861755453);
#2219=CYLINDRICAL_SURFACE('',#2527,0.124032861755453);
#2220=CYLINDRICAL_SURFACE('',#2534,0.749041401963156);
#2221=CYLINDRICAL_SURFACE('',#2536,0.124032861755453);
#2222=CYLINDRICAL_SURFACE('',#2538,0.124032861755453);
#2223=CYLINDRICAL_SURFACE('',#2545,0.749041401963155);
#2224=CYLINDRICAL_SURFACE('',#2547,0.124032861755453);
#2225=CYLINDRICAL_SURFACE('',#2549,0.124032861755453);
#2226=CYLINDRICAL_SURFACE('',#2556,0.749041401963156);
#2227=CYLINDRICAL_SURFACE('',#2558,0.124032861755453);
#2228=CYLINDRICAL_SURFACE('',#2560,0.124032861755453);
#2229=CYLINDRICAL_SURFACE('',#2567,0.749041401963156);
#2230=CYLINDRICAL_SURFACE('',#2569,0.124032861755453);
#2231=CYLINDRICAL_SURFACE('',#2571,0.124032861755453);
#2232=CYLINDRICAL_SURFACE('',#2578,0.749041401963155);
#2233=CYLINDRICAL_SURFACE('',#2580,0.124032861755453);
#2234=CYLINDRICAL_SURFACE('',#2582,0.124032861755453);
#2235=CYLINDRICAL_SURFACE('',#2589,0.749041401963156);
#2236=CYLINDRICAL_SURFACE('',#2591,0.124032861755453);
#2237=CYLINDRICAL_SURFACE('',#2593,0.124032861755453);
#2238=CYLINDRICAL_SURFACE('',#2600,0.749041401963155);
#2239=CYLINDRICAL_SURFACE('',#2602,0.124032861755453);
#2240=CYLINDRICAL_SURFACE('',#2604,4.75930776765241);
#2241=CYLINDRICAL_SURFACE('',#2623,0.124032861755453);
#2242=CYLINDRICAL_SURFACE('',#2629,0.749041401963155);
#2243=CYLINDRICAL_SURFACE('',#2631,0.124032861755453);
#2244=CYLINDRICAL_SURFACE('',#2639,6.94701057265674);
#2245=CYLINDRICAL_SURFACE('',#2664,6.94665463816359);
#2274=ADVANCED_FACE('',(#245),#2195,.F.);
#2275=ADVANCED_FACE('',(#246),#2196,.F.);
#2276=ADVANCED_FACE('',(#247),#2197,.F.);
#2277=ADVANCED_FACE('',(#248),#2198,.T.);
#2278=ADVANCED_FACE('',(#249),#58,.F.);
#2279=ADVANCED_FACE('',(#250),#2199,.F.);
#2280=ADVANCED_FACE('',(#251),#2200,.T.);
#2281=ADVANCED_FACE('',(#252),#2201,.T.);
#2282=ADVANCED_FACE('',(#253),#59,.F.);
#2283=ADVANCED_FACE('',(#254),#2202,.F.);
#2284=ADVANCED_FACE('',(#255),#2203,.T.);
#2285=ADVANCED_FACE('',(#256),#2204,.T.);
#2286=ADVANCED_FACE('',(#257),#60,.F.);
#2287=ADVANCED_FACE('',(#258),#2205,.F.);
#2288=ADVANCED_FACE('',(#259),#2206,.T.);
#2289=ADVANCED_FACE('',(#260),#2207,.T.);
#2290=ADVANCED_FACE('',(#261),#61,.F.);
#2291=ADVANCED_FACE('',(#262),#2208,.F.);
#2292=ADVANCED_FACE('',(#263),#2209,.T.);
#2293=ADVANCED_FACE('',(#264),#2210,.T.);
#2294=ADVANCED_FACE('',(#265),#62,.F.);
#2295=ADVANCED_FACE('',(#266),#2211,.F.);
#2296=ADVANCED_FACE('',(#267),#2212,.T.);
#2297=ADVANCED_FACE('',(#268),#2213,.T.);
#2298=ADVANCED_FACE('',(#269),#63,.F.);
#2299=ADVANCED_FACE('',(#270),#2214,.F.);
#2300=ADVANCED_FACE('',(#271),#2215,.T.);
#2301=ADVANCED_FACE('',(#272),#2216,.T.);
#2302=ADVANCED_FACE('',(#273),#64,.F.);
#2303=ADVANCED_FACE('',(#274),#2217,.F.);
#2304=ADVANCED_FACE('',(#275),#2218,.T.);
#2305=ADVANCED_FACE('',(#276),#2219,.T.);
#2306=ADVANCED_FACE('',(#277),#65,.F.);
#2307=ADVANCED_FACE('',(#278),#2220,.F.);
#2308=ADVANCED_FACE('',(#279),#2221,.T.);
#2309=ADVANCED_FACE('',(#280),#2222,.T.);
#2310=ADVANCED_FACE('',(#281),#66,.F.);
#2311=ADVANCED_FACE('',(#282),#2223,.F.);
#2312=ADVANCED_FACE('',(#283),#2224,.T.);
#2313=ADVANCED_FACE('',(#284),#2225,.T.);
#2314=ADVANCED_FACE('',(#285),#67,.F.);
#2315=ADVANCED_FACE('',(#286),#2226,.F.);
#2316=ADVANCED_FACE('',(#287),#2227,.T.);
#2317=ADVANCED_FACE('',(#288),#2228,.T.);
#2318=ADVANCED_FACE('',(#289),#68,.F.);
#2319=ADVANCED_FACE('',(#290),#2229,.F.);
#2320=ADVANCED_FACE('',(#291),#2230,.T.);
#2321=ADVANCED_FACE('',(#292),#2231,.T.);
#2322=ADVANCED_FACE('',(#293),#69,.F.);
#2323=ADVANCED_FACE('',(#294),#2232,.F.);
#2324=ADVANCED_FACE('',(#295),#2233,.T.);
#2325=ADVANCED_FACE('',(#296),#2234,.T.);
#2326=ADVANCED_FACE('',(#297),#70,.F.);
#2327=ADVANCED_FACE('',(#298),#2235,.F.);
#2328=ADVANCED_FACE('',(#299),#2236,.T.);
#2329=ADVANCED_FACE('',(#300),#2237,.T.);
#2330=ADVANCED_FACE('',(#301),#71,.F.);
#2331=ADVANCED_FACE('',(#302),#2238,.F.);
#2332=ADVANCED_FACE('',(#303),#2239,.T.);
#2333=ADVANCED_FACE('',(#304),#2240,.T.);
#2334=ADVANCED_FACE('',(#305),#2241,.T.);
#2335=ADVANCED_FACE('',(#306),#72,.F.);
#2336=ADVANCED_FACE('',(#307),#2242,.F.);
#2337=ADVANCED_FACE('',(#308),#2243,.T.);
#2338=ADVANCED_FACE('',(#309,#49),#73,.T.);
#2339=ADVANCED_FACE('',(#310,#50),#74,.T.);
#2340=ADVANCED_FACE('',(#311),#39,.T.);
#2341=ADVANCED_FACE('',(#312,#51),#2244,.T.);
#2342=ADVANCED_FACE('',(#313),#40,.T.);
#2343=ADVANCED_FACE('',(#314,#52),#75,.T.);
#2344=ADVANCED_FACE('',(#315),#41,.F.);
#2345=ADVANCED_FACE('',(#316),#42,.T.);
#2346=ADVANCED_FACE('',(#317,#53),#76,.T.);
#2347=ADVANCED_FACE('',(#318),#43,.F.);
#2348=ADVANCED_FACE('',(#319),#44,.F.);
#2349=ADVANCED_FACE('',(#320,#54),#77,.T.);
#2350=ADVANCED_FACE('',(#321),#45,.T.);
#2351=ADVANCED_FACE('',(#322),#46,.F.);
#2352=ADVANCED_FACE('',(#323,#55),#78,.T.);
#2353=ADVANCED_FACE('',(#324),#47,.T.);
#2354=ADVANCED_FACE('',(#325),#2245,.T.);
#2355=ADVANCED_FACE('',(#326),#48,.T.);
#2406=CLOSED_SHELL('',(#2274,#2275,#2276,#2277,#2278,#2279,#2280,#2281,
#2282,#2283,#2284,#2285,#2286,#2287,#2288,#2289,#2290,#2291,#2292,#2293,
#2294,#2295,#2296,#2297,#2298,#2299,#2300,#2301,#2302,#2303,#2304,#2305,
#2306,#2307,#2308,#2309,#2310,#2311,#2312,#2313,#2314,#2315,#2316,#2317,
#2318,#2319,#2320,#2321,#2322,#2323,#2324,#2325,#2326,#2327,#2328,#2329,
#2330,#2331,#2332,#2333,#2334,#2335,#2336,#2337,#2338,#2339,#2340,#2341,
#2342,#2343,#2344,#2345,#2346,#2347,#2348,#2349,#2350,#2351,#2352,#2353,
#2354,#2355));
#2444=AXIS2_PLACEMENT_3D('',#3431,#2728,#2729);
#2445=AXIS2_PLACEMENT_3D('',#3432,#2730,#2731);
#2446=AXIS2_PLACEMENT_3D('',#3525,#2733,#2734);
#2447=AXIS2_PLACEMENT_3D('',#3527,#2735,#2736);
#2448=AXIS2_PLACEMENT_3D('',#3558,#2739,#2740);
#2449=AXIS2_PLACEMENT_3D('',#3575,#2741,#2742);
#2450=AXIS2_PLACEMENT_3D('',#3618,#2744,#2745);
#2451=AXIS2_PLACEMENT_3D('',#3623,#2747,#2748);
#2452=AXIS2_PLACEMENT_3D('',#3626,#2750,#2751);
#2453=AXIS2_PLACEMENT_3D('',#3627,#2752,#2753);
#2454=AXIS2_PLACEMENT_3D('',#3629,#2754,#2755);
#2455=AXIS2_PLACEMENT_3D('',#3631,#2756,#2757);
#2456=AXIS2_PLACEMENT_3D('',#3632,#2758,#2759);
#2457=AXIS2_PLACEMENT_3D('',#3633,#2760,#2761);
#2458=AXIS2_PLACEMENT_3D('',#3635,#2762,#2763);
#2459=AXIS2_PLACEMENT_3D('',#3637,#2765,#2766);
#2460=AXIS2_PLACEMENT_3D('',#3640,#2768,#2769);
#2461=AXIS2_PLACEMENT_3D('',#3641,#2770,#2771);
#2462=AXIS2_PLACEMENT_3D('',#3646,#2773,#2774);
#2463=AXIS2_PLACEMENT_3D('',#3649,#2776,#2777);
#2464=AXIS2_PLACEMENT_3D('',#3650,#2778,#2779);
#2465=AXIS2_PLACEMENT_3D('',#3652,#2780,#2781);
#2466=AXIS2_PLACEMENT_3D('',#3654,#2782,#2783);
#2467=AXIS2_PLACEMENT_3D('',#3655,#2784,#2785);
#2468=AXIS2_PLACEMENT_3D('',#3656,#2786,#2787);
#2469=AXIS2_PLACEMENT_3D('',#3658,#2788,#2789);
#2470=AXIS2_PLACEMENT_3D('',#3660,#2791,#2792);
#2471=AXIS2_PLACEMENT_3D('',#3663,#2794,#2795);
#2472=AXIS2_PLACEMENT_3D('',#3664,#2796,#2797);
#2473=AXIS2_PLACEMENT_3D('',#3669,#2799,#2800);
#2474=AXIS2_PLACEMENT_3D('',#3672,#2802,#2803);
#2475=AXIS2_PLACEMENT_3D('',#3673,#2804,#2805);
#2476=AXIS2_PLACEMENT_3D('',#3675,#2806,#2807);
#2477=AXIS2_PLACEMENT_3D('',#3677,#2808,#2809);
#2478=AXIS2_PLACEMENT_3D('',#3678,#2810,#2811);
#2479=AXIS2_PLACEMENT_3D('',#3679,#2812,#2813);
#2480=AXIS2_PLACEMENT_3D('',#3681,#2814,#2815);
#2481=AXIS2_PLACEMENT_3D('',#3683,#2817,#2818);
#2482=AXIS2_PLACEMENT_3D('',#3686,#2820,#2821);
#2483=AXIS2_PLACEMENT_3D('',#3687,#2822,#2823);
#2484=AXIS2_PLACEMENT_3D('',#3692,#2825,#2826);
#2485=AXIS2_PLACEMENT_3D('',#3695,#2828,#2829);
#2486=AXIS2_PLACEMENT_3D('',#3696,#2830,#2831);
#2487=AXIS2_PLACEMENT_3D('',#3698,#2832,#2833);
#2488=AXIS2_PLACEMENT_3D('',#3700,#2834,#2835);
#2489=AXIS2_PLACEMENT_3D('',#3701,#2836,#2837);
#2490=AXIS2_PLACEMENT_3D('',#3702,#2838,#2839);
#2491=AXIS2_PLACEMENT_3D('',#3704,#2840,#2841);
#2492=AXIS2_PLACEMENT_3D('',#3706,#2843,#2844);
#2493=AXIS2_PLACEMENT_3D('',#3709,#2846,#2847);
#2494=AXIS2_PLACEMENT_3D('',#3710,#2848,#2849);
#2495=AXIS2_PLACEMENT_3D('',#3715,#2851,#2852);
#2496=AXIS2_PLACEMENT_3D('',#3718,#2854,#2855);
#2497=AXIS2_PLACEMENT_3D('',#3719,#2856,#2857);
#2498=AXIS2_PLACEMENT_3D('',#3721,#2858,#2859);
#2499=AXIS2_PLACEMENT_3D('',#3723,#2860,#2861);
#2500=AXIS2_PLACEMENT_3D('',#3724,#2862,#2863);
#2501=AXIS2_PLACEMENT_3D('',#3725,#2864,#2865);
#2502=AXIS2_PLACEMENT_3D('',#3727,#2866,#2867);
#2503=AXIS2_PLACEMENT_3D('',#3729,#2869,#2870);
#2504=AXIS2_PLACEMENT_3D('',#3732,#2872,#2873);
#2505=AXIS2_PLACEMENT_3D('',#3733,#2874,#2875);
#2506=AXIS2_PLACEMENT_3D('',#3738,#2877,#2878);
#2507=AXIS2_PLACEMENT_3D('',#3741,#2880,#2881);
#2508=AXIS2_PLACEMENT_3D('',#3742,#2882,#2883);
#2509=AXIS2_PLACEMENT_3D('',#3744,#2884,#2885);
#2510=AXIS2_PLACEMENT_3D('',#3746,#2886,#2887);
#2511=AXIS2_PLACEMENT_3D('',#3747,#2888,#2889);
#2512=AXIS2_PLACEMENT_3D('',#3748,#2890,#2891);
#2513=AXIS2_PLACEMENT_3D('',#3750,#2892,#2893);
#2514=AXIS2_PLACEMENT_3D('',#3752,#2895,#2896);
#2515=AXIS2_PLACEMENT_3D('',#3755,#2898,#2899);
#2516=AXIS2_PLACEMENT_3D('',#3756,#2900,#2901);
#2517=AXIS2_PLACEMENT_3D('',#3761,#2903,#2904);
#2518=AXIS2_PLACEMENT_3D('',#3764,#2906,#2907);
#2519=AXIS2_PLACEMENT_3D('',#3765,#2908,#2909);
#2520=AXIS2_PLACEMENT_3D('',#3767,#2910,#2911);
#2521=AXIS2_PLACEMENT_3D('',#3769,#2912,#2913);
#2522=AXIS2_PLACEMENT_3D('',#3770,#2914,#2915);
#2523=AXIS2_PLACEMENT_3D('',#3771,#2916,#2917);
#2524=AXIS2_PLACEMENT_3D('',#3773,#2918,#2919);
#2525=AXIS2_PLACEMENT_3D('',#3775,#2921,#2922);
#2526=AXIS2_PLACEMENT_3D('',#3778,#2924,#2925);
#2527=AXIS2_PLACEMENT_3D('',#3779,#2926,#2927);
#2528=AXIS2_PLACEMENT_3D('',#3784,#2929,#2930);
#2529=AXIS2_PLACEMENT_3D('',#3787,#2932,#2933);
#2530=AXIS2_PLACEMENT_3D('',#3788,#2934,#2935);
#2531=AXIS2_PLACEMENT_3D('',#3790,#2936,#2937);
#2532=AXIS2_PLACEMENT_3D('',#3792,#2938,#2939);
#2533=AXIS2_PLACEMENT_3D('',#3793,#2940,#2941);
#2534=AXIS2_PLACEMENT_3D('',#3794,#2942,#2943);
#2535=AXIS2_PLACEMENT_3D('',#3796,#2944,#2945);
#2536=AXIS2_PLACEMENT_3D('',#3798,#2947,#2948);
#2537=AXIS2_PLACEMENT_3D('',#3801,#2950,#2951);
#2538=AXIS2_PLACEMENT_3D('',#3802,#2952,#2953);
#2539=AXIS2_PLACEMENT_3D('',#3807,#2955,#2956);
#2540=AXIS2_PLACEMENT_3D('',#3810,#2958,#2959);
#2541=AXIS2_PLACEMENT_3D('',#3811,#2960,#2961);
#2542=AXIS2_PLACEMENT_3D('',#3813,#2962,#2963);
#2543=AXIS2_PLACEMENT_3D('',#3815,#2964,#2965);
#2544=AXIS2_PLACEMENT_3D('',#3816,#2966,#2967);
#2545=AXIS2_PLACEMENT_3D('',#3817,#2968,#2969);
#2546=AXIS2_PLACEMENT_3D('',#3819,#2970,#2971);
#2547=AXIS2_PLACEMENT_3D('',#3821,#2973,#2974);
#2548=AXIS2_PLACEMENT_3D('',#3824,#2976,#2977);
#2549=AXIS2_PLACEMENT_3D('',#3825,#2978,#2979);
#2550=AXIS2_PLACEMENT_3D('',#3830,#2981,#2982);
#2551=AXIS2_PLACEMENT_3D('',#3833,#2984,#2985);
#2552=AXIS2_PLACEMENT_3D('',#3834,#2986,#2987);
#2553=AXIS2_PLACEMENT_3D('',#3836,#2988,#2989);
#2554=AXIS2_PLACEMENT_3D('',#3838,#2990,#2991);
#2555=AXIS2_PLACEMENT_3D('',#3839,#2992,#2993);
#2556=AXIS2_PLACEMENT_3D('',#3840,#2994,#2995);
#2557=AXIS2_PLACEMENT_3D('',#3842,#2996,#2997);
#2558=AXIS2_PLACEMENT_3D('',#3844,#2999,#3000);
#2559=AXIS2_PLACEMENT_3D('',#3847,#3002,#3003);
#2560=AXIS2_PLACEMENT_3D('',#3848,#3004,#3005);
#2561=AXIS2_PLACEMENT_3D('',#3853,#3007,#3008);
#2562=AXIS2_PLACEMENT_3D('',#3856,#3010,#3011);
#2563=AXIS2_PLACEMENT_3D('',#3857,#3012,#3013);
#2564=AXIS2_PLACEMENT_3D('',#3859,#3014,#3015);
#2565=AXIS2_PLACEMENT_3D('',#3861,#3016,#3017);
#2566=AXIS2_PLACEMENT_3D('',#3862,#3018,#3019);
#2567=AXIS2_PLACEMENT_3D('',#3863,#3020,#3021);
#2568=AXIS2_PLACEMENT_3D('',#3865,#3022,#3023);
#2569=AXIS2_PLACEMENT_3D('',#3867,#3025,#3026);
#2570=AXIS2_PLACEMENT_3D('',#3870,#3028,#3029);
#2571=AXIS2_PLACEMENT_3D('',#3871,#3030,#3031);
#2572=AXIS2_PLACEMENT_3D('',#3876,#3033,#3034);
#2573=AXIS2_PLACEMENT_3D('',#3879,#3036,#3037);
#2574=AXIS2_PLACEMENT_3D('',#3880,#3038,#3039);
#2575=AXIS2_PLACEMENT_3D('',#3882,#3040,#3041);
#2576=AXIS2_PLACEMENT_3D('',#3884,#3042,#3043);
#2577=AXIS2_PLACEMENT_3D('',#3885,#3044,#3045);
#2578=AXIS2_PLACEMENT_3D('',#3886,#3046,#3047);
#2579=AXIS2_PLACEMENT_3D('',#3888,#3048,#3049);
#2580=AXIS2_PLACEMENT_3D('',#3890,#3051,#3052);
#2581=AXIS2_PLACEMENT_3D('',#3893,#3054,#3055);
#2582=AXIS2_PLACEMENT_3D('',#3894,#3056,#3057);
#2583=AXIS2_PLACEMENT_3D('',#3899,#3059,#3060);
#2584=AXIS2_PLACEMENT_3D('',#3902,#3062,#3063);
#2585=AXIS2_PLACEMENT_3D('',#3903,#3064,#3065);
#2586=AXIS2_PLACEMENT_3D('',#3905,#3066,#3067);
#2587=AXIS2_PLACEMENT_3D('',#3907,#3068,#3069);
#2588=AXIS2_PLACEMENT_3D('',#3908,#3070,#3071);
#2589=AXIS2_PLACEMENT_3D('',#3909,#3072,#3073);
#2590=AXIS2_PLACEMENT_3D('',#3911,#3074,#3075);
#2591=AXIS2_PLACEMENT_3D('',#3913,#3077,#3078);
#2592=AXIS2_PLACEMENT_3D('',#3916,#3080,#3081);
#2593=AXIS2_PLACEMENT_3D('',#3917,#3082,#3083);
#2594=AXIS2_PLACEMENT_3D('',#3922,#3085,#3086);
#2595=AXIS2_PLACEMENT_3D('',#3925,#3088,#3089);
#2596=AXIS2_PLACEMENT_3D('',#3926,#3090,#3091);
#2597=AXIS2_PLACEMENT_3D('',#3928,#3092,#3093);
#2598=AXIS2_PLACEMENT_3D('',#3930,#3094,#3095);
#2599=AXIS2_PLACEMENT_3D('',#3931,#3096,#3097);
#2600=AXIS2_PLACEMENT_3D('',#3932,#3098,#3099);
#2601=AXIS2_PLACEMENT_3D('',#3934,#3100,#3101);
#2602=AXIS2_PLACEMENT_3D('',#3936,#3103,#3104);
#2603=AXIS2_PLACEMENT_3D('',#3939,#3106,#3107);
#2604=AXIS2_PLACEMENT_3D('',#3940,#3108,#3109);
#2605=AXIS2_PLACEMENT_3D('',#3943,#3110,#3111);
#2606=AXIS2_PLACEMENT_3D('',#3946,#3113,#3114);
#2607=AXIS2_PLACEMENT_3D('',#3948,#3115,#3116);
#2608=AXIS2_PLACEMENT_3D('',#3951,#3118,#3119);
#2609=AXIS2_PLACEMENT_3D('',#3952,#3120,#3121);
#2610=AXIS2_PLACEMENT_3D('',#3953,#3122,#3123);
#2611=AXIS2_PLACEMENT_3D('',#3954,#3124,#3125);
#2612=AXIS2_PLACEMENT_3D('',#3955,#3126,#3127);
#2613=AXIS2_PLACEMENT_3D('',#3956,#3128,#3129);
#2614=AXIS2_PLACEMENT_3D('',#3957,#3130,#3131);
#2615=AXIS2_PLACEMENT_3D('',#3958,#3132,#3133);
#2616=AXIS2_PLACEMENT_3D('',#3959,#3134,#3135);
#2617=AXIS2_PLACEMENT_3D('',#3960,#3136,#3137);
#2618=AXIS2_PLACEMENT_3D('',#3961,#3138,#3139);
#2619=AXIS2_PLACEMENT_3D('',#3962,#3140,#3141);
#2620=AXIS2_PLACEMENT_3D('',#3963,#3142,#3143);
#2621=AXIS2_PLACEMENT_3D('',#3964,#3144,#3145);
#2622=AXIS2_PLACEMENT_3D('',#3966,#3146,#3147);
#2623=AXIS2_PLACEMENT_3D('',#3968,#3149,#3150);
#2624=AXIS2_PLACEMENT_3D('',#3970,#3151,#3152);
#2625=AXIS2_PLACEMENT_3D('',#3973,#3154,#3155);
#2626=AXIS2_PLACEMENT_3D('',#3974,#3156,#3157);
#2627=AXIS2_PLACEMENT_3D('',#3976,#3158,#3159);
#2628=AXIS2_PLACEMENT_3D('',#3977,#3160,#3161);
#2629=AXIS2_PLACEMENT_3D('',#3978,#3162,#3163);
#2630=AXIS2_PLACEMENT_3D('',#3980,#3164,#3165);
#2631=AXIS2_PLACEMENT_3D('',#3982,#3167,#3168);
#2632=AXIS2_PLACEMENT_3D('',#3983,#3169,#3170);
#2633=AXIS2_PLACEMENT_3D('',#3984,#3171,#3172);
#2634=AXIS2_PLACEMENT_3D('',#3986,#3173,#3174);
#2635=AXIS2_PLACEMENT_3D('',#3987,#3175,#3176);
#2636=AXIS2_PLACEMENT_3D('',#3989,#3177,#3178);
#2637=AXIS2_PLACEMENT_3D('',#3990,#3179,#3180);
#2638=AXIS2_PLACEMENT_3D('',#3992,#3181,#3182);
#2639=AXIS2_PLACEMENT_3D('',#3994,#3184,#3185);
#2640=AXIS2_PLACEMENT_3D('',#3996,#3186,#3187);
#2641=AXIS2_PLACEMENT_3D('',#3999,#3190,#3191);
#2642=AXIS2_PLACEMENT_3D('',#4002,#3193,#3194);
#2643=AXIS2_PLACEMENT_3D('',#4003,#3195,#3196);
#2644=AXIS2_PLACEMENT_3D('',#4005,#3197,#3198);
#2645=AXIS2_PLACEMENT_3D('',#4006,#3199,#3200);
#2646=AXIS2_PLACEMENT_3D('',#4008,#3201,#3202);
#2647=AXIS2_PLACEMENT_3D('',#4010,#3204,#3205);
#2648=AXIS2_PLACEMENT_3D('',#4013,#3207,#3208);
#2649=AXIS2_PLACEMENT_3D('',#4014,#3209,#3210);
#2650=AXIS2_PLACEMENT_3D('',#4016,#3211,#3212);
#2651=AXIS2_PLACEMENT_3D('',#4017,#3213,#3214);
#2652=AXIS2_PLACEMENT_3D('',#4019,#3216,#3217);
#2653=AXIS2_PLACEMENT_3D('',#4022,#3219,#3220);
#2654=AXIS2_PLACEMENT_3D('',#4023,#3221,#3222);
#2655=AXIS2_PLACEMENT_3D('',#4025,#3223,#3224);
#2656=AXIS2_PLACEMENT_3D('',#4026,#3225,#3226);
#2657=AXIS2_PLACEMENT_3D('',#4028,#3227,#3228);
#2658=AXIS2_PLACEMENT_3D('',#4030,#3230,#3231);
#2659=AXIS2_PLACEMENT_3D('',#4033,#3233,#3234);
#2660=AXIS2_PLACEMENT_3D('',#4034,#3235,#3236);
#2661=AXIS2_PLACEMENT_3D('',#4036,#3237,#3238);
#2662=AXIS2_PLACEMENT_3D('',#4037,#3239,#3240);
#2663=AXIS2_PLACEMENT_3D('',#4039,#3241,#3242);
#2664=AXIS2_PLACEMENT_3D('',#4041,#3244,#3245);
#2665=AXIS2_PLACEMENT_3D('',#4043,#3246,#3247);
#2666=AXIS2_PLACEMENT_3D('',#4045,#3249,#3250);
#2728=DIRECTION('axis',(0.,0.,1.));
#2729=DIRECTION('refdir',(1.,0.,0.));
#2730=DIRECTION('center_axis',(0.,1.,0.));
#2731=DIRECTION('ref_axis',(1.,0.,0.));
#2732=DIRECTION('',(0.,1.,0.));
#2733=DIRECTION('center_axis',(0.,0.,-1.));
#2734=DIRECTION('ref_axis',(-1.,0.,0.));
#2735=DIRECTION('center_axis',(0.,0.,-1.));
#2736=DIRECTION('ref_axis',(1.,0.,0.));
#2737=DIRECTION('',(0.,0.,-1.));
#2738=DIRECTION('',(0.,0.,-1.));
#2739=DIRECTION('center_axis',(0.,0.,-1.));
#2740=DIRECTION('ref_axis',(1.,0.,0.));
#2741=DIRECTION('center_axis',(1.,0.,0.));
#2742=DIRECTION('ref_axis',(0.,1.,0.));
#2743=DIRECTION('',(1.,0.,0.));
#2744=DIRECTION('center_axis',(0.,0.,1.));
#2745=DIRECTION('ref_axis',(0.975941703326222,0.218031630064795,0.));
#2746=DIRECTION('',(0.,0.,1.));
#2747=DIRECTION('center_axis',(0.,0.,1.));
#2748=DIRECTION('ref_axis',(0.975941703326222,0.218031630064795,0.));
#2749=DIRECTION('',(0.,0.,1.));
#2750=DIRECTION('center_axis',(0.,0.,-1.));
#2751=DIRECTION('ref_axis',(0.975941703326222,0.218031630064795,0.));
#2752=DIRECTION('center_axis',(0.,0.,1.));
#2753=DIRECTION('ref_axis',(-0.913545457642601,-0.406736643075801,0.));
#2754=DIRECTION('center_axis',(0.,0.,1.));
#2755=DIRECTION('ref_axis',(-1.,0.,0.));
#2756=DIRECTION('center_axis',(0.,0.,1.));
#2757=DIRECTION('ref_axis',(-0.611669535952668,0.791113379224146,0.));
#2758=DIRECTION('center_axis',(0.,0.,-1.));
#2759=DIRECTION('ref_axis',(0.591883195117478,-0.806023748618815,0.));
#2760=DIRECTION('center_axis',(0.,0.,1.));
#2761=DIRECTION('ref_axis',(-0.611669535952668,0.791113379224146,0.));
#2762=DIRECTION('center_axis',(0.,0.,1.));
#2763=DIRECTION('ref_axis',(-0.611669535952668,0.791113379224146,0.));
#2764=DIRECTION('',(0.,0.,1.));
#2765=DIRECTION('center_axis',(0.,0.,1.));
#2766=DIRECTION('ref_axis',(0.591883195117478,-0.806023748618815,0.));
#2767=DIRECTION('',(0.,0.,-1.));
#2768=DIRECTION('center_axis',(0.,0.,1.));
#2769=DIRECTION('ref_axis',(0.591883195117478,-0.806023748618815,0.));
#2770=DIRECTION('center_axis',(0.,0.,1.));
#2771=DIRECTION('ref_axis',(0.802885656700754,0.596133057516692,0.));
#2772=DIRECTION('',(0.,0.,1.));
#2773=DIRECTION('center_axis',(0.,0.,1.));
#2774=DIRECTION('ref_axis',(0.802885656700754,0.596133057516692,0.));
#2775=DIRECTION('',(0.,0.,1.));
#2776=DIRECTION('center_axis',(0.,0.,-1.));
#2777=DIRECTION('ref_axis',(0.802885656700754,0.596133057516692,0.));
#2778=DIRECTION('center_axis',(0.,0.,1.));
#2779=DIRECTION('ref_axis',(-0.669130606358858,-0.743144825477395,0.));
#2780=DIRECTION('center_axis',(0.,0.,1.));
#2781=DIRECTION('ref_axis',(-1.,0.,0.));
#2782=DIRECTION('center_axis',(0.,0.,1.));
#2783=DIRECTION('ref_axis',(-0.880562726305899,0.473929620345386,0.));
#2784=DIRECTION('center_axis',(0.,0.,-1.));
#2785=DIRECTION('ref_axis',(0.86855159810715,-0.495598750427718,0.));
#2786=DIRECTION('center_axis',(0.,0.,1.));
#2787=DIRECTION('ref_axis',(-0.880562726305899,0.473929620345386,0.));
#2788=DIRECTION('center_axis',(0.,0.,1.));
#2789=DIRECTION('ref_axis',(-0.880562726305899,0.473929620345386,0.));
#2790=DIRECTION('',(0.,0.,1.));
#2791=DIRECTION('center_axis',(0.,0.,1.));
#2792=DIRECTION('ref_axis',(0.86855159810715,-0.495598750427718,0.));
#2793=DIRECTION('',(0.,0.,-1.));
#2794=DIRECTION('center_axis',(0.,0.,1.));
#2795=DIRECTION('ref_axis',(0.86855159810715,-0.495598750427718,0.));
#2796=DIRECTION('center_axis',(0.,0.,1.));
#2797=DIRECTION('ref_axis',(0.491003386044519,0.871157663625143,0.));
#2798=DIRECTION('',(0.,0.,1.));
#2799=DIRECTION('center_axis',(0.,0.,1.));
#2800=DIRECTION('ref_axis',(0.491003386044519,0.871157663625143,0.));
#2801=DIRECTION('',(0.,0.,1.));
#2802=DIRECTION('center_axis',(0.,0.,-1.));
#2803=DIRECTION('ref_axis',(0.491003386044519,0.871157663625143,0.));
#2804=DIRECTION('center_axis',(0.,0.,1.));
#2805=DIRECTION('ref_axis',(-0.309016994374947,-0.951056516295154,0.));
#2806=DIRECTION('center_axis',(0.,0.,1.));
#2807=DIRECTION('ref_axis',(-1.,0.,0.));
#2808=DIRECTION('center_axis',(0.,0.,1.));
#2809=DIRECTION('ref_axis',(-0.99719862161961,0.0747991245934742,0.));
#2810=DIRECTION('center_axis',(0.,0.,-1.));
#2811=DIRECTION('ref_axis',(0.99503953924054,-0.0994802259143675,0.));
#2812=DIRECTION('center_axis',(0.,0.,1.));
#2813=DIRECTION('ref_axis',(-0.99719862161961,0.0747991245934742,0.));
#2814=DIRECTION('center_axis',(0.,0.,1.));
#2815=DIRECTION('ref_axis',(-0.99719862161961,0.0747991245934742,0.));
#2816=DIRECTION('',(0.,0.,1.));
#2817=DIRECTION('center_axis',(0.,0.,1.));
#2818=DIRECTION('ref_axis',(0.99503953924054,-0.0994802259143675,0.));
#2819=DIRECTION('',(0.,0.,-1.));
#2820=DIRECTION('center_axis',(0.,0.,1.));
#2821=DIRECTION('ref_axis',(0.99503953924054,-0.0994802259143675,0.));
#2822=DIRECTION('center_axis',(0.,0.,1.));
#2823=DIRECTION('ref_axis',(0.0942221693154581,0.995551195473889,0.));
#2824=DIRECTION('',(0.,0.,1.));
#2825=DIRECTION('center_axis',(0.,0.,1.));
#2826=DIRECTION('ref_axis',(0.0942221693154581,0.995551195473889,0.));
#2827=DIRECTION('',(0.,0.,1.));
#2828=DIRECTION('center_axis',(0.,0.,-1.));
#2829=DIRECTION('ref_axis',(0.0942221693154581,0.995551195473889,0.));
#2830=DIRECTION('center_axis',(0.,0.,1.));
#2831=DIRECTION('ref_axis',(0.104528463267654,-0.994521895368273,0.));
#2832=DIRECTION('center_axis',(0.,0.,1.));
#2833=DIRECTION('ref_axis',(-1.,0.,0.));
#2834=DIRECTION('center_axis',(0.,0.,1.));
#2835=DIRECTION('ref_axis',(-0.941409815990215,-0.337264819329364,0.));
#2836=DIRECTION('center_axis',(0.,0.,-1.));
#2837=DIRECTION('ref_axis',(0.949476104388814,0.313839333409058,0.));
#2838=DIRECTION('center_axis',(0.,0.,1.));
#2839=DIRECTION('ref_axis',(-0.941409815990215,-0.337264819329364,0.));
#2840=DIRECTION('center_axis',(0.,0.,1.));
#2841=DIRECTION('ref_axis',(-0.941409815990215,-0.337264819329364,0.));
#2842=DIRECTION('',(0.,0.,1.));
#2843=DIRECTION('center_axis',(0.,0.,1.));
#2844=DIRECTION('ref_axis',(0.949476104388814,0.313839333409058,0.));
#2845=DIRECTION('',(0.,0.,-1.));
#2846=DIRECTION('center_axis',(0.,0.,1.));
#2847=DIRECTION('ref_axis',(0.949476104388814,0.313839333409058,0.));
#2848=DIRECTION('center_axis',(0.,0.,1.));
#2849=DIRECTION('ref_axis',(-0.31885091646978,0.947804881326521,0.));
#2850=DIRECTION('',(0.,0.,1.));
#2851=DIRECTION('center_axis',(0.,0.,1.));
#2852=DIRECTION('ref_axis',(-0.31885091646978,0.947804881326521,0.));
#2853=DIRECTION('',(0.,0.,1.));
#2854=DIRECTION('center_axis',(0.,0.,-1.));
#2855=DIRECTION('ref_axis',(-0.31885091646978,0.947804881326521,0.));
#2856=DIRECTION('center_axis',(0.,0.,1.));
#2857=DIRECTION('ref_axis',(0.5,-0.866025403784438,0.));
#2858=DIRECTION('center_axis',(0.,0.,1.));
#2859=DIRECTION('ref_axis',(-1.,0.,0.));
#2860=DIRECTION('center_axis',(0.,0.,1.));
#2861=DIRECTION('ref_axis',(-0.722842700736426,-0.69101261203546,0.));
#2862=DIRECTION('center_axis',(0.,0.,-1.));
#2863=DIRECTION('ref_axis',(0.739739625368646,0.672893220845221,0.));
#2864=DIRECTION('center_axis',(0.,0.,1.));
#2865=DIRECTION('ref_axis',(-0.722842700736426,-0.69101261203546,0.));
#2866=DIRECTION('center_axis',(0.,0.,1.));
#2867=DIRECTION('ref_axis',(-0.722842700736426,-0.69101261203546,0.));
#2868=DIRECTION('',(0.,0.,1.));
#2869=DIRECTION('center_axis',(0.,0.,1.));
#2870=DIRECTION('ref_axis',(0.739739625368646,0.672893220845221,0.));
#2871=DIRECTION('',(0.,0.,-1.));
#2872=DIRECTION('center_axis',(0.,0.,1.));
#2873=DIRECTION('ref_axis',(0.739739625368646,0.672893220845221,0.));
#2874=DIRECTION('center_axis',(0.,0.,1.));
#2875=DIRECTION('ref_axis',(-0.676791782127754,0.736174492660767,0.));
#2876=DIRECTION('',(0.,0.,1.));
#2877=DIRECTION('center_axis',(0.,0.,1.));
#2878=DIRECTION('ref_axis',(-0.676791782127754,0.736174492660767,0.));
#2879=DIRECTION('',(0.,0.,1.));
#2880=DIRECTION('center_axis',(0.,0.,-1.));
#2881=DIRECTION('ref_axis',(-0.676791782127754,0.736174492660767,0.));
#2882=DIRECTION('center_axis',(0.,0.,1.));
#2883=DIRECTION('ref_axis',(0.809016994374948,-0.587785252292473,0.));
#2884=DIRECTION('center_axis',(0.,0.,1.));
#2885=DIRECTION('ref_axis',(-1.,0.,0.));
#2886=DIRECTION('center_axis',(0.,0.,1.));
#2887=DIRECTION('ref_axis',(-0.379289515705529,-0.925278046468123,0.));
#2888=DIRECTION('center_axis',(0.,0.,-1.));
#2889=DIRECTION('ref_axis',(0.402095444798718,0.915597757354244,0.));
#2890=DIRECTION('center_axis',(0.,0.,1.));
#2891=DIRECTION('ref_axis',(-0.379289515705529,-0.925278046468123,0.));
#2892=DIRECTION('center_axis',(0.,0.,1.));
#2893=DIRECTION('ref_axis',(-0.379289515705529,-0.925278046468123,0.));
#2894=DIRECTION('',(0.,0.,1.));
#2895=DIRECTION('center_axis',(0.,0.,1.));
#2896=DIRECTION('ref_axis',(0.402095444798718,0.915597757354244,0.));
#2897=DIRECTION('',(0.,0.,-1.));
#2898=DIRECTION('center_axis',(0.,0.,1.));
#2899=DIRECTION('ref_axis',(0.402095444798718,0.915597757354244,0.));
#2900=DIRECTION('center_axis',(0.,0.,1.));
#2901=DIRECTION('ref_axis',(-0.917709200195522,0.397252846278659,0.));
#2902=DIRECTION('',(0.,0.,1.));
#2903=DIRECTION('center_axis',(0.,0.,1.));
#2904=DIRECTION('ref_axis',(-0.917709200195522,0.397252846278659,0.));
#2905=DIRECTION('',(0.,0.,1.));
#2906=DIRECTION('center_axis',(0.,0.,-1.));
#2907=DIRECTION('ref_axis',(-0.917709200195522,0.397252846278659,0.));
#2908=DIRECTION('center_axis',(0.,0.,1.));
#2909=DIRECTION('ref_axis',(0.978147600733806,-0.207911690817759,0.));
#2910=DIRECTION('center_axis',(0.,0.,1.));
#2911=DIRECTION('ref_axis',(-1.,0.,0.));
#2912=DIRECTION('center_axis',(0.,0.,1.));
#2913=DIRECTION('ref_axis',(0.0298462723279306,-0.999554500779286,0.));
#2914=DIRECTION('center_axis',(0.,0.,-1.));
#2915=DIRECTION('ref_axis',(-0.00507469109934694,0.999987123672223,0.));
#2916=DIRECTION('center_axis',(0.,0.,1.));
#2917=DIRECTION('ref_axis',(0.0298462723279306,-0.999554500779286,0.));
#2918=DIRECTION('center_axis',(0.,0.,1.));
#2919=DIRECTION('ref_axis',(0.0298462723279306,-0.999554500779286,0.));
#2920=DIRECTION('',(0.,0.,1.));
#2921=DIRECTION('center_axis',(0.,0.,1.));
#2922=DIRECTION('ref_axis',(-0.00507469109934694,0.999987123672223,0.));
#2923=DIRECTION('',(0.,0.,-1.));
#2924=DIRECTION('center_axis',(0.,0.,1.));
#2925=DIRECTION('ref_axis',(-0.00507469109934694,0.999987123672223,0.));
#2926=DIRECTION('center_axis',(0.,0.,1.));
#2927=DIRECTION('ref_axis',(-0.999946360423132,-0.0103574261538407,0.));
#2928=DIRECTION('',(0.,0.,1.));
#2929=DIRECTION('center_axis',(0.,0.,1.));
#2930=DIRECTION('ref_axis',(-0.999946360423132,-0.0103574261538407,0.));
#2931=DIRECTION('',(0.,0.,1.));
#2932=DIRECTION('center_axis',(0.,0.,-1.));
#2933=DIRECTION('ref_axis',(-0.999946360423132,-0.0103574261538407,0.));
#2934=DIRECTION('center_axis',(0.,0.,1.));
#2935=DIRECTION('ref_axis',(0.978147600733805,0.20791169081776,0.));
#2936=DIRECTION('center_axis',(0.,0.,1.));
#2937=DIRECTION('ref_axis',(-1.,0.,0.));
#2938=DIRECTION('center_axis',(0.,0.,1.));
#2939=DIRECTION('ref_axis',(0.433821368731019,-0.900998901238145,0.));
#2940=DIRECTION('center_axis',(0.,0.,-1.));
#2941=DIRECTION('ref_axis',(-0.411367366804213,0.911469631709454,0.));
#2942=DIRECTION('center_axis',(0.,0.,1.));
#2943=DIRECTION('ref_axis',(0.433821368731019,-0.900998901238145,0.));
#2944=DIRECTION('center_axis',(0.,0.,1.));
#2945=DIRECTION('ref_axis',(0.433821368731019,-0.900998901238145,0.));
#2946=DIRECTION('',(0.,0.,1.));
#2947=DIRECTION('center_axis',(0.,0.,1.));
#2948=DIRECTION('ref_axis',(-0.411367366804213,0.911469631709454,0.));
#2949=DIRECTION('',(0.,0.,-1.));
#2950=DIRECTION('center_axis',(0.,0.,1.));
#2951=DIRECTION('ref_axis',(-0.411367366804213,0.911469631709454,0.));
#2952=DIRECTION('center_axis',(0.,0.,1.));
#2953=DIRECTION('ref_axis',(-0.909283710706085,-0.416176805510078,0.));
#2954=DIRECTION('',(0.,0.,1.));
#2955=DIRECTION('center_axis',(0.,0.,1.));
#2956=DIRECTION('ref_axis',(-0.909283710706085,-0.416176805510078,0.));
#2957=DIRECTION('',(0.,0.,1.));
#2958=DIRECTION('center_axis',(0.,0.,-1.));
#2959=DIRECTION('ref_axis',(-0.909283710706085,-0.416176805510078,0.));
#2960=DIRECTION('center_axis',(0.,0.,1.));
#2961=DIRECTION('ref_axis',(0.809016994374947,0.587785252292473,0.));
#2962=DIRECTION('center_axis',(0.,0.,1.));
#2963=DIRECTION('ref_axis',(-1.,0.,0.));
#2964=DIRECTION('center_axis',(0.,0.,1.));
#2965=DIRECTION('ref_axis',(0.762784809337106,-0.646652406354879,0.));
#2966=DIRECTION('center_axis',(0.,0.,-1.));
#2967=DIRECTION('ref_axis',(-0.746530887633426,0.66535075998247,0.));
#2968=DIRECTION('center_axis',(0.,0.,1.));
#2969=DIRECTION('ref_axis',(0.762784809337106,-0.646652406354879,0.));
#2970=DIRECTION('center_axis',(0.,0.,1.));
#2971=DIRECTION('ref_axis',(0.762784809337106,-0.646652406354879,0.));
#2972=DIRECTION('',(0.,0.,1.));
#2973=DIRECTION('center_axis',(0.,0.,1.));
#2974=DIRECTION('ref_axis',(-0.746530887633426,0.66535075998247,0.));
#2975=DIRECTION('',(0.,0.,-1.));
#2976=DIRECTION('center_axis',(0.,0.,1.));
#2977=DIRECTION('ref_axis',(-0.746530887633426,0.66535075998247,0.));
#2978=DIRECTION('center_axis',(0.,0.,1.));
#2979=DIRECTION('ref_axis',(-0.661397646824773,-0.75003543434604,0.));
#2980=DIRECTION('',(0.,0.,1.));
#2981=DIRECTION('center_axis',(0.,0.,1.));
#2982=DIRECTION('ref_axis',(-0.661397646824773,-0.75003543434604,0.));
#2983=DIRECTION('',(0.,0.,1.));
#2984=DIRECTION('center_axis',(0.,0.,-1.));
#2985=DIRECTION('ref_axis',(-0.661397646824773,-0.75003543434604,0.));
#2986=DIRECTION('center_axis',(0.,0.,1.));
#2987=DIRECTION('ref_axis',(0.5,0.866025403784439,0.));
#2988=DIRECTION('center_axis',(0.,0.,1.));
#2989=DIRECTION('ref_axis',(-1.,0.,0.));
#2990=DIRECTION('center_axis',(0.,0.,1.));
#2991=DIRECTION('ref_axis',(0.959855826726362,-0.280493835760168,0.));
#2992=DIRECTION('center_axis',(0.,0.,-1.));
#2993=DIRECTION('ref_axis',(-0.952612435970617,0.30418669733262,0.));
#2994=DIRECTION('center_axis',(0.,0.,1.));
#2995=DIRECTION('ref_axis',(0.959855826726362,-0.280493835760168,0.));
#2996=DIRECTION('center_axis',(0.,0.,1.));
#2997=DIRECTION('ref_axis',(0.959855826726362,-0.280493835760168,0.));
#2998=DIRECTION('',(0.,0.,1.));
#2999=DIRECTION('center_axis',(0.,0.,1.));
#3000=DIRECTION('ref_axis',(-0.952612435970617,0.30418669733262,0.));
#3001=DIRECTION('',(0.,0.,-1.));
#3002=DIRECTION('center_axis',(0.,0.,1.));
#3003=DIRECTION('ref_axis',(-0.952612435970617,0.30418669733262,0.));
#3004=DIRECTION('center_axis',(0.,0.,1.));
#3005=DIRECTION('ref_axis',(-0.299149921198468,-0.954206122725562,0.));
#3006=DIRECTION('',(0.,0.,1.));
#3007=DIRECTION('center_axis',(0.,0.,1.));
#3008=DIRECTION('ref_axis',(-0.299149921198468,-0.954206122725562,0.));
#3009=DIRECTION('',(0.,0.,1.));
#3010=DIRECTION('center_axis',(0.,0.,-1.));
#3011=DIRECTION('ref_axis',(-0.299149921198468,-0.954206122725562,0.));
#3012=DIRECTION('center_axis',(0.,0.,1.));
#3013=DIRECTION('ref_axis',(0.104528463267653,0.994521895368273,0.));
#3014=DIRECTION('center_axis',(0.,0.,1.));
#3015=DIRECTION('ref_axis',(-1.,0.,0.));
#3016=DIRECTION('center_axis',(0.,0.,1.));
#3017=DIRECTION('ref_axis',(0.990959051658197,0.134164667243976,0.));
#3018=DIRECTION('center_axis',(0.,0.,-1.));
#3019=DIRECTION('ref_axis',(-0.993978639916195,-0.109574008735429,0.));
#3020=DIRECTION('center_axis',(0.,0.,1.));
#3021=DIRECTION('ref_axis',(0.990959051658197,0.134164667243976,0.));
#3022=DIRECTION('center_axis',(0.,0.,1.));
#3023=DIRECTION('ref_axis',(0.990959051658197,0.134164667243976,0.));
#3024=DIRECTION('',(0.,0.,1.));
#3025=DIRECTION('center_axis',(0.,0.,1.));
#3026=DIRECTION('ref_axis',(-0.993978639916195,-0.109574008735429,0.));
#3027=DIRECTION('',(0.,0.,-1.));
#3028=DIRECTION('center_axis',(0.,0.,1.));
#3029=DIRECTION('ref_axis',(-0.993978639916195,-0.109574008735429,0.));
#3030=DIRECTION('center_axis',(0.,0.,1.));
#3031=DIRECTION('ref_axis',(0.114823543494768,-0.99338590379535,0.));
#3032=DIRECTION('',(0.,0.,1.));
#3033=DIRECTION('center_axis',(0.,0.,1.));
#3034=DIRECTION('ref_axis',(0.114823543494768,-0.99338590379535,0.));
#3035=DIRECTION('',(0.,0.,1.));
#3036=DIRECTION('center_axis',(0.,0.,-1.));
#3037=DIRECTION('ref_axis',(0.114823543494768,-0.99338590379535,0.));
#3038=DIRECTION('center_axis',(0.,0.,1.));
#3039=DIRECTION('ref_axis',(-0.309016994374947,0.951056516295154,0.));
#3040=DIRECTION('center_axis',(0.,0.,1.));
#3041=DIRECTION('ref_axis',(-1.,0.,0.));
#3042=DIRECTION('center_axis',(0.,0.,1.));
#3043=DIRECTION('ref_axis',(0.850716453977969,0.525624880433899,0.));
#3044=DIRECTION('center_axis',(0.,0.,-1.));
#3045=DIRECTION('ref_axis',(-0.863476907007803,-0.504388373244505,0.));
#3046=DIRECTION('center_axis',(0.,0.,1.));
#3047=DIRECTION('ref_axis',(0.850716453977969,0.525624880433899,0.));
#3048=DIRECTION('center_axis',(0.,0.,1.));
#3049=DIRECTION('ref_axis',(0.850716453977969,0.525624880433899,0.));
#3050=DIRECTION('',(0.,0.,1.));
#3051=DIRECTION('center_axis',(0.,0.,1.));
#3052=DIRECTION('ref_axis',(-0.863476907007803,-0.504388373244505,0.));
#3053=DIRECTION('',(0.,0.,-1.));
#3054=DIRECTION('center_axis',(0.,0.,1.));
#3055=DIRECTION('ref_axis',(-0.863476907007803,-0.504388373244505,0.));
#3056=DIRECTION('center_axis',(0.,0.,1.));
#3057=DIRECTION('ref_axis',(0.508942974378613,-0.860800237471302,0.));
#3058=DIRECTION('',(0.,0.,1.));
#3059=DIRECTION('center_axis',(0.,0.,1.));
#3060=DIRECTION('ref_axis',(0.508942974378613,-0.860800237471302,0.));
#3061=DIRECTION('',(0.,0.,1.));
#3062=DIRECTION('center_axis',(0.,0.,-1.));
#3063=DIRECTION('ref_axis',(0.508942974378613,-0.860800237471302,0.));
#3064=DIRECTION('center_axis',(0.,0.,1.));
#3065=DIRECTION('ref_axis',(-0.669130606358858,0.743144825477394,0.));
#3066=DIRECTION('center_axis',(0.,0.,1.));
#3067=DIRECTION('ref_axis',(-1.,0.,0.));
#3068=DIRECTION('center_axis',(0.,0.,1.));
#3069=DIRECTION('ref_axis',(0.563377252888591,0.826199776644671,0.));
#3070=DIRECTION('center_axis',(0.,0.,-1.));
#3071=DIRECTION('ref_axis',(-0.583672172436327,-0.811989405795087,0.));
#3072=DIRECTION('center_axis',(0.,0.,1.));
#3073=DIRECTION('ref_axis',(0.563377252888591,0.826199776644671,0.));
#3074=DIRECTION('center_axis',(0.,0.,1.));
#3075=DIRECTION('ref_axis',(0.563377252888591,0.826199776644671,0.));
#3076=DIRECTION('',(0.,0.,1.));
#3077=DIRECTION('center_axis',(0.,0.,1.));
#3078=DIRECTION('ref_axis',(-0.583672172436327,-0.811989405795087,0.));
#3079=DIRECTION('',(0.,0.,-1.));
#3080=DIRECTION('center_axis',(0.,0.,1.));
#3081=DIRECTION('ref_axis',(-0.583672172436327,-0.811989405795087,0.));
#3082=DIRECTION('center_axis',(0.,0.,1.));
#3083=DIRECTION('ref_axis',(0.815061541390626,-0.57937438996381,0.));
#3084=DIRECTION('',(0.,0.,1.));
#3085=DIRECTION('center_axis',(0.,0.,1.));
#3086=DIRECTION('ref_axis',(0.815061541390626,-0.57937438996381,0.));
#3087=DIRECTION('',(0.,0.,1.));
#3088=DIRECTION('center_axis',(0.,0.,-1.));
#3089=DIRECTION('ref_axis',(0.815061541390626,-0.57937438996381,0.));
#3090=DIRECTION('center_axis',(0.,0.,1.));
#3091=DIRECTION('ref_axis',(-0.913545457642601,0.4067366430758,0.));
#3092=DIRECTION('center_axis',(0.,0.,1.));
#3093=DIRECTION('ref_axis',(-1.,0.,0.));
#3094=DIRECTION('center_axis',(0.,0.,1.));
#3095=DIRECTION('ref_axis',(0.17862500665311,0.983917225684242,0.));
#3096=DIRECTION('center_axis',(0.,0.,-1.));
#3097=DIRECTION('ref_axis',(-0.202945216755389,-0.979190093391528,0.));
#3098=DIRECTION('center_axis',(0.,0.,1.));
#3099=DIRECTION('ref_axis',(0.17862500665311,0.983917225684242,0.));
#3100=DIRECTION('center_axis',(0.,0.,1.));
#3101=DIRECTION('ref_axis',(0.17862500665311,0.983917225684242,0.));
#3102=DIRECTION('',(0.,0.,1.));
#3103=DIRECTION('center_axis',(0.,0.,1.));
#3104=DIRECTION('ref_axis',(-0.202945216755389,-0.979190093391528,0.));
#3105=DIRECTION('',(0.,0.,-1.));
#3106=DIRECTION('center_axis',(0.,0.,1.));
#3107=DIRECTION('ref_axis',(-0.202945216755389,-0.979190093391528,0.));
#3108=DIRECTION('center_axis',(0.,0.,-1.));
#3109=DIRECTION('ref_axis',(-1.,0.,0.));
#3110=DIRECTION('center_axis',(0.,0.,1.));
#3111=DIRECTION('ref_axis',(-1.,0.,0.));
#3112=DIRECTION('',(0.,0.,1.));
#3113=DIRECTION('center_axis',(0.,0.,-1.));
#3114=DIRECTION('ref_axis',(1.,0.,0.));
#3115=DIRECTION('center_axis',(0.,0.,1.));
#3116=DIRECTION('ref_axis',(-1.,0.,0.));
#3117=DIRECTION('',(0.,0.,-1.));
#3118=DIRECTION('center_axis',(0.,0.,-1.));
#3119=DIRECTION('ref_axis',(1.,0.,0.));
#3120=DIRECTION('center_axis',(0.,0.,-1.));
#3121=DIRECTION('ref_axis',(1.,0.,0.));
#3122=DIRECTION('center_axis',(0.,0.,-1.));
#3123=DIRECTION('ref_axis',(1.,0.,0.));
#3124=DIRECTION('center_axis',(0.,0.,-1.));
#3125=DIRECTION('ref_axis',(1.,0.,0.));
#3126=DIRECTION('center_axis',(0.,0.,-1.));
#3127=DIRECTION('ref_axis',(1.,0.,0.));
#3128=DIRECTION('center_axis',(0.,0.,-1.));
#3129=DIRECTION('ref_axis',(1.,0.,0.));
#3130=DIRECTION('center_axis',(0.,0.,-1.));
#3131=DIRECTION('ref_axis',(1.,0.,0.));
#3132=DIRECTION('center_axis',(0.,0.,-1.));
#3133=DIRECTION('ref_axis',(1.,0.,0.));
#3134=DIRECTION('center_axis',(0.,0.,-1.));
#3135=DIRECTION('ref_axis',(1.,0.,0.));
#3136=DIRECTION('center_axis',(0.,0.,-1.));
#3137=DIRECTION('ref_axis',(1.,0.,0.));
#3138=DIRECTION('center_axis',(0.,0.,-1.));
#3139=DIRECTION('ref_axis',(1.,0.,0.));
#3140=DIRECTION('center_axis',(0.,0.,-1.));
#3141=DIRECTION('ref_axis',(1.,0.,0.));
#3142=DIRECTION('center_axis',(0.,0.,-1.));
#3143=DIRECTION('ref_axis',(1.,0.,0.));
#3144=DIRECTION('center_axis',(0.,0.,-1.));
#3145=DIRECTION('ref_axis',(1.,0.,0.));
#3146=DIRECTION('center_axis',(0.,0.,-1.));
#3147=DIRECTION('ref_axis',(1.,0.,0.));
#3148=DIRECTION('',(0.,0.,1.));
#3149=DIRECTION('center_axis',(0.,0.,1.));
#3150=DIRECTION('ref_axis',(0.980248563294553,-0.197769446980481,0.));
#3151=DIRECTION('center_axis',(0.,0.,1.));
#3152=DIRECTION('ref_axis',(0.980248563294553,-0.197769446980481,0.));
#3153=DIRECTION('',(0.,0.,1.));
#3154=DIRECTION('center_axis',(0.,0.,-1.));
#3155=DIRECTION('ref_axis',(0.980248563294553,-0.197769446980481,0.));
#3156=DIRECTION('center_axis',(0.,0.,1.));
#3157=DIRECTION('ref_axis',(-1.,0.,0.));
#3158=DIRECTION('center_axis',(0.,0.,1.));
#3159=DIRECTION('ref_axis',(-0.237013125989935,0.971506447795628,0.));
#3160=DIRECTION('center_axis',(0.,0.,-1.));
#3161=DIRECTION('ref_axis',(0.212872810601971,-0.977079918177841,0.));
#3162=DIRECTION('center_axis',(0.,0.,1.));
#3163=DIRECTION('ref_axis',(-0.237013125989935,0.971506447795628,0.));
#3164=DIRECTION('center_axis',(0.,0.,1.));
#3165=DIRECTION('ref_axis',(-0.237013125989935,0.971506447795628,0.));
#3166=DIRECTION('',(0.,0.,1.));
#3167=DIRECTION('center_axis',(0.,0.,1.));
#3168=DIRECTION('ref_axis',(0.212872810601971,-0.977079918177841,0.));
#3169=DIRECTION('center_axis',(0.,0.,1.));
#3170=DIRECTION('ref_axis',(0.212872810601971,-0.977079918177841,0.));
#3171=DIRECTION('center_axis',(0.,0.,-1.));
#3172=DIRECTION('ref_axis',(-1.,0.,0.));
#3173=DIRECTION('center_axis',(0.,0.,-1.));
#3174=DIRECTION('ref_axis',(1.,0.,0.));
#3175=DIRECTION('center_axis',(0.,0.,1.));
#3176=DIRECTION('ref_axis',(1.,0.,0.));
#3177=DIRECTION('center_axis',(0.,0.,-1.));
#3178=DIRECTION('ref_axis',(1.,0.,0.));
#3179=DIRECTION('center_axis',(0.,0.,-1.));
#3180=DIRECTION('ref_axis',(-1.,0.,0.));
#3181=DIRECTION('center_axis',(0.,0.,-1.));
#3182=DIRECTION('ref_axis',(1.,0.,0.));
#3183=DIRECTION('',(-0.709089650734988,8.68384371081118E-17,0.705118335615046));
#3184=DIRECTION('center_axis',(0.,0.,-1.));
#3185=DIRECTION('ref_axis',(-1.,0.,0.));
#3186=DIRECTION('center_axis',(0.,0.,-1.));
#3187=DIRECTION('ref_axis',(1.,0.,0.));
#3188=DIRECTION('',(0.,0.,1.));
#3189=DIRECTION('',(0.,0.,1.));
#3190=DIRECTION('center_axis',(0.,0.,1.));
#3191=DIRECTION('ref_axis',(-1.,0.,0.));
#3192=DIRECTION('',(-0.705118335615046,-8.63520912731075E-17,-0.709089650734988));
#3193=DIRECTION('center_axis',(0.,0.,-1.));
#3194=DIRECTION('ref_axis',(1.,0.,0.));
#3195=DIRECTION('center_axis',(0.,0.,-1.));
#3196=DIRECTION('ref_axis',(-1.,0.,0.));
#3197=DIRECTION('center_axis',(0.,0.,-1.));
#3198=DIRECTION('ref_axis',(1.,0.,0.));
#3199=DIRECTION('center_axis',(0.,0.,-1.));
#3200=DIRECTION('ref_axis',(-1.,0.,0.));
#3201=DIRECTION('center_axis',(0.,0.,-1.));
#3202=DIRECTION('ref_axis',(1.,0.,0.));
#3203=DIRECTION('',(0.799712036156634,-9.79364785318835E-17,-0.600383759962084));
#3204=DIRECTION('center_axis',(0.,0.,1.));
#3205=DIRECTION('ref_axis',(-1.,0.,0.));
#3206=DIRECTION('',(-0.795904561203624,-9.74701973304796E-17,-0.605422108495608));
#3207=DIRECTION('center_axis',(0.,0.,-1.));
#3208=DIRECTION('ref_axis',(1.,0.,0.));
#3209=DIRECTION('center_axis',(0.,0.,-1.));
#3210=DIRECTION('ref_axis',(-1.,0.,0.));
#3211=DIRECTION('center_axis',(0.,0.,-1.));
#3212=DIRECTION('ref_axis',(1.,0.,0.));
#3213=DIRECTION('center_axis',(0.,0.,-1.));
#3214=DIRECTION('ref_axis',(-1.,0.,0.));
#3215=DIRECTION('',(0.710031613960551,-8.69537943330218E-17,-0.704169799960617));
#3216=DIRECTION('center_axis',(0.,0.,1.));
#3217=DIRECTION('ref_axis',(-1.,0.,0.));
#3218=DIRECTION('',(0.704169799960617,8.62359291578001E-17,0.710031613960551));
#3219=DIRECTION('center_axis',(0.,0.,-1.));
#3220=DIRECTION('ref_axis',(1.,0.,0.));
#3221=DIRECTION('center_axis',(0.,0.,1.));
#3222=DIRECTION('ref_axis',(1.,0.,0.));
#3223=DIRECTION('center_axis',(0.,0.,-1.));
#3224=DIRECTION('ref_axis',(1.,0.,0.));
#3225=DIRECTION('center_axis',(0.,0.,-1.));
#3226=DIRECTION('ref_axis',(-1.,0.,0.));
#3227=DIRECTION('center_axis',(0.,0.,-1.));
#3228=DIRECTION('ref_axis',(1.,0.,0.));
#3229=DIRECTION('',(-0.790648054928562,9.68264609720345E-17,0.612270898571605));
#3230=DIRECTION('center_axis',(0.,0.,1.));
#3231=DIRECTION('ref_axis',(-1.,0.,0.));
#3232=DIRECTION('',(0.802697028722426,9.8302034691001E-17,0.596387022058821));
#3233=DIRECTION('center_axis',(0.,0.,-1.));
#3234=DIRECTION('ref_axis',(1.,0.,0.));
#3235=DIRECTION('center_axis',(0.,0.,1.));
#3236=DIRECTION('ref_axis',(1.,0.,0.));
#3237=DIRECTION('center_axis',(0.,0.,-1.));
#3238=DIRECTION('ref_axis',(1.,0.,0.));
#3239=DIRECTION('center_axis',(0.,0.,-1.));
#3240=DIRECTION('ref_axis',(-1.,0.,0.));
#3241=DIRECTION('center_axis',(0.,0.,-1.));
#3242=DIRECTION('ref_axis',(1.,0.,0.));
#3243=DIRECTION('',(-0.699050213581169,8.56089606505452E-17,0.715072582953732));
#3244=DIRECTION('center_axis',(0.,0.,-1.));
#3245=DIRECTION('ref_axis',(-1.,0.,0.));
#3246=DIRECTION('center_axis',(0.,0.,-1.));
#3247=DIRECTION('ref_axis',(1.,0.,0.));
#3248=DIRECTION('',(0.,0.,1.));
#3249=DIRECTION('center_axis',(0.,0.,1.));
#3250=DIRECTION('ref_axis',(-1.,0.,0.));
#3251=DIRECTION('',(-0.715072582953733,-8.75711349872319E-17,-0.699050213581168));
#3431=CARTESIAN_POINT('',(0.,0.,0.));
#3432=CARTESIAN_POINT('Origin',(0.,0.,3.64730359255819));
#3433=CARTESIAN_POINT('',(1.7686229373189,1.76804321859845,2.71234996365709));
#3434=CARTESIAN_POINT('',(-2.00054127207588,1.50061272066065,3.64730359255819));
#3435=CARTESIAN_POINT('Ctrl Pts',(1.76862293715133,1.76804321917473,2.7123499640497));
#3436=CARTESIAN_POINT('Ctrl Pts',(1.67326196575883,1.86343545816792,2.53195855620751));
#3437=CARTESIAN_POINT('Ctrl Pts',(1.55118349747322,1.96856998381331,2.36929449097458));
#3438=CARTESIAN_POINT('Ctrl Pts',(1.246000460916,2.17790854658287,2.06411145441735));
#3439=CARTESIAN_POINT('Ctrl Pts',(1.02949498881865,2.29363907921209,1.91141759608479));
#3440=CARTESIAN_POINT('Ctrl Pts',(0.539267048392588,2.45557152312544,1.70247672387608));
#3441=CARTESIAN_POINT('Ctrl Pts',(0.26499702638238,2.50080065552765,1.64676232048231));
#3442=CARTESIAN_POINT('Ctrl Pts',(-0.26499702638238,2.50080065552765,1.64676232048231));
#3443=CARTESIAN_POINT('Ctrl Pts',(-0.539267048392587,2.45557152312544,1.70247672387608));
#3444=CARTESIAN_POINT('Ctrl Pts',(-1.02949498881865,2.29363907921209,1.91141759608479));
#3445=CARTESIAN_POINT('Ctrl Pts',(-1.246000460916,2.17790854658287,2.06411145441735));
#3446=CARTESIAN_POINT('Ctrl Pts',(-1.58860233127999,1.94290274824875,2.40671332478134));
#3447=CARTESIAN_POINT('Ctrl Pts',(-1.73834101649832,1.80421211541924,2.62302156240085));
#3448=CARTESIAN_POINT('Ctrl Pts',(-1.89232803732295,1.6367193793479,2.98513719870131));
#3449=CARTESIAN_POINT('Ctrl Pts',(-1.93234128425375,1.58804832718918,3.11227541726051));
#3450=CARTESIAN_POINT('Ctrl Pts',(-1.98643480897785,1.51987885041677,3.37495601917005));
#3451=CARTESIAN_POINT('Ctrl Pts',(-2.00054127207588,1.50061272066065,3.51055323926873));
#3452=CARTESIAN_POINT('Ctrl Pts',(-2.00054127207588,1.50061272066065,3.64730359255819));
#3453=CARTESIAN_POINT('',(1.76857489436387,1.76809127600101,4.58234809718318));
#3454=CARTESIAN_POINT('Ctrl Pts',(1.76857489410945,1.76809127582596,4.5823480969561));
#3455=CARTESIAN_POINT('Ctrl Pts',(1.79165762592203,1.79117807736387,4.53868863499553));
#3456=CARTESIAN_POINT('Ctrl Pts',(1.81337315467134,1.81289707546748,4.49369536588909));
#3457=CARTESIAN_POINT('Ctrl Pts',(1.88690002208923,1.88643457058566,4.32522974835823));
#3458=CARTESIAN_POINT('Ctrl Pts',(1.92922149639063,1.92875988806683,4.19441050122833));
#3459=CARTESIAN_POINT('Ctrl Pts',(1.98603528459668,1.9855745276702,3.92446964748283));
#3460=CARTESIAN_POINT('Ctrl Pts',(2.00053500325065,2.00007126058529,3.78535115919203));
#3461=CARTESIAN_POINT('Ctrl Pts',(2.00054753639194,2.00007126058529,3.50944616688294));
#3462=CARTESIAN_POINT('Ctrl Pts',(1.98606217458304,1.98557625302193,3.37033412466248));
#3463=CARTESIAN_POINT('Ctrl Pts',(1.92927930620037,1.92876635631918,3.10040251938398));
#3464=CARTESIAN_POINT('Ctrl Pts',(1.88697439789821,1.88644406872771,2.96958607054619));
#3465=CARTESIAN_POINT('Ctrl Pts',(1.8134528306885,1.81289198848806,2.8010799828847));
#3466=CARTESIAN_POINT('Ctrl Pts',(1.79172259628398,1.79115269770373,2.7560468766317));
#3467=CARTESIAN_POINT('Ctrl Pts',(1.76862293706403,1.76804321842309,2.71234996388456));
#3468=CARTESIAN_POINT('Ctrl Pts',(-2.00054127207588,1.50061272066065,3.64730359255819));
#3469=CARTESIAN_POINT('Ctrl Pts',(-2.00054127207588,1.50061272066065,3.78405394584766));
#3470=CARTESIAN_POINT('Ctrl Pts',(-1.98643480897785,1.51987885041677,3.91965116594633));
#3471=CARTESIAN_POINT('Ctrl Pts',(-1.93234128425375,1.58804832718918,4.18233176785587));
#3472=CARTESIAN_POINT('Ctrl Pts',(-1.89232803732295,1.6367193793479,4.30946998641508));
#3473=CARTESIAN_POINT('Ctrl Pts',(-1.73834101649832,1.80421211541924,4.67158562271553));
#3474=CARTESIAN_POINT('Ctrl Pts',(-1.58860233127999,1.94290274824875,4.88789386033504));
#3475=CARTESIAN_POINT('Ctrl Pts',(-1.246000460916,2.17790854658287,5.23049573069903));
#3476=CARTESIAN_POINT('Ctrl Pts',(-1.02949498881865,2.29363907921209,5.38318958903159));
#3477=CARTESIAN_POINT('Ctrl Pts',(-0.539267048392588,2.45557152312544,5.5921304612403));
#3478=CARTESIAN_POINT('Ctrl Pts',(-0.26499702638238,2.50080065552765,5.64784486463407));
#3479=CARTESIAN_POINT('Ctrl Pts',(0.264997026382379,2.50080065552765,5.64784486463407));
#3480=CARTESIAN_POINT('Ctrl Pts',(0.539267048392587,2.45557152312544,5.5921304612403));
#3481=CARTESIAN_POINT('Ctrl Pts',(1.02949498881865,2.29363907921209,5.38318958903159));
#3482=CARTESIAN_POINT('Ctrl Pts',(1.246000460916,2.17790854658287,5.23049573069903));
#3483=CARTESIAN_POINT('Ctrl Pts',(1.55116056163378,1.96858571652152,4.92533562998125));
#3484=CARTESIAN_POINT('Ctrl Pts',(1.67322122242047,1.86347102998993,4.76270326620755));
#3485=CARTESIAN_POINT('Ctrl Pts',(1.76857489419661,1.76809127657624,4.58234809679125));
#3486=CARTESIAN_POINT('',(-2.00054127207588,6.65272805060642,3.64730359255819));
#3487=CARTESIAN_POINT('',(-2.00054127207588,0.,3.64730359255819));
#3488=CARTESIAN_POINT('',(2.00054127207588,6.65272805060642,3.64730359255819));
#3489=CARTESIAN_POINT('Ctrl Pts',(2.00054127207588,6.65272805060642,3.64730359255819));
#3490=CARTESIAN_POINT('Ctrl Pts',(2.00054127207588,6.65272805060642,3.90007910394674));
#3491=CARTESIAN_POINT('Ctrl Pts',(1.94972968142331,6.66864085099173,4.168651787778));
#3492=CARTESIAN_POINT('Ctrl Pts',(1.74514049605878,6.7250799896849,4.66107620583205));
#3493=CARTESIAN_POINT('Ctrl Pts',(1.59143342856617,6.76468178320297,4.88506276304886));
#3494=CARTESIAN_POINT('Ctrl Pts',(1.23780358335032,6.83823119596726,5.23869260826471));
#3495=CARTESIAN_POINT('Ctrl Pts',(1.01379886205209,6.87710358589666,5.39243413099089));
#3496=CARTESIAN_POINT('Ctrl Pts',(0.521308842207693,6.93185249060457,5.59704867604272));
#3497=CARTESIAN_POINT('Ctrl Pts',(0.25271202651198,6.94701057265674,5.64784486463407));
#3498=CARTESIAN_POINT('Ctrl Pts',(-0.25271202651198,6.94701057265674,5.64784486463407));
#3499=CARTESIAN_POINT('Ctrl Pts',(-0.521308842207694,6.93185249060457,5.59704867604272));
#3500=CARTESIAN_POINT('Ctrl Pts',(-1.01379886205209,6.87710358589666,5.39243413099088));
#3501=CARTESIAN_POINT('Ctrl Pts',(-1.23780358335032,6.83823119596726,5.23869260826471));
#3502=CARTESIAN_POINT('Ctrl Pts',(-1.59143342856617,6.76468178320297,4.88506276304886));
#3503=CARTESIAN_POINT('Ctrl Pts',(-1.74514049605878,6.7250799896849,4.66107620583205));
#3504=CARTESIAN_POINT('Ctrl Pts',(-1.94972968142331,6.66864085099173,4.168651787778));
#3505=CARTESIAN_POINT('Ctrl Pts',(-2.00054127207588,6.65272805060642,3.90007910394674));
#3506=CARTESIAN_POINT('Ctrl Pts',(-2.00054127207588,6.65272805060642,3.64730359255819));
#3507=CARTESIAN_POINT('Ctrl Pts',(-2.00054127207588,6.65272805060642,3.64730359255819));
#3508=CARTESIAN_POINT('Ctrl Pts',(-2.00054127207588,6.65272805060642,3.39452808116964));
#3509=CARTESIAN_POINT('Ctrl Pts',(-1.94972968142331,6.66864085099173,3.12595539733838));
#3510=CARTESIAN_POINT('Ctrl Pts',(-1.74514049605878,6.7250799896849,2.63353097928433));
#3511=CARTESIAN_POINT('Ctrl Pts',(-1.59143342856617,6.76468178320297,2.40954442206752));
#3512=CARTESIAN_POINT('Ctrl Pts',(-1.23780358335032,6.83823119596726,2.05591457685167));
#3513=CARTESIAN_POINT('Ctrl Pts',(-1.01379886205209,6.87710358589666,1.9021730541255));
#3514=CARTESIAN_POINT('Ctrl Pts',(-0.521308842207694,6.93185249060457,1.69755850907366));
#3515=CARTESIAN_POINT('Ctrl Pts',(-0.25271202651198,6.94701057265674,1.64676232048231));
#3516=CARTESIAN_POINT('Ctrl Pts',(0.25271202651198,6.94701057265674,1.64676232048231));
#3517=CARTESIAN_POINT('Ctrl Pts',(0.521308842207693,6.93185249060457,1.69755850907366));
#3518=CARTESIAN_POINT('Ctrl Pts',(1.01379886205209,6.87710358589666,1.9021730541255));
#3519=CARTESIAN_POINT('Ctrl Pts',(1.23780358335032,6.83823119596726,2.05591457685167));
#3520=CARTESIAN_POINT('Ctrl Pts',(1.59143342856617,6.76468178320297,2.40954442206752));
#3521=CARTESIAN_POINT('Ctrl Pts',(1.74514049605878,6.7250799896849,2.63353097928433));
#3522=CARTESIAN_POINT('Ctrl Pts',(1.94972968142331,6.66864085099173,3.12595539733838));
#3523=CARTESIAN_POINT('Ctrl Pts',(2.00054127207588,6.65272805060642,3.39452808116964));
#3524=CARTESIAN_POINT('Ctrl Pts',(2.00054127207588,6.65272805060642,3.64730359255819));
#3525=CARTESIAN_POINT('Origin',(0.,0.,7.74376865817678));
#3526=CARTESIAN_POINT('',(2.50080065552765,-3.06259751809754E-16,15.268401777045));
#3527=CARTESIAN_POINT('Origin',(0.,0.,15.268401777045));
#3528=CARTESIAN_POINT('',(2.50080065552765,-1.43519978267323E-17,5.64746572886916));
#3529=CARTESIAN_POINT('',(2.50080065552765,-3.06259751809754E-16,7.74376865817678));
#3530=CARTESIAN_POINT('',(1.50123911195662,-2.00007126058529,3.64739446828387));
#3531=CARTESIAN_POINT('Ctrl Pts',(2.50080065552765,2.77555756156289E-16,
5.64746572886916));
#3532=CARTESIAN_POINT('Ctrl Pts',(2.50080065552765,-0.264926868087175,5.64746572886916));
#3533=CARTESIAN_POINT('Ctrl Pts',(2.45559485322071,-0.539128651599931,5.59176763614851));
#3534=CARTESIAN_POINT('Ctrl Pts',(2.29374488883448,-1.02924237889175,5.38287897435064));
#3535=CARTESIAN_POINT('Ctrl Pts',(2.1780735274369,-1.24570166067483,5.23022071004141));
#3536=CARTESIAN_POINT('Ctrl Pts',(1.94320134506485,-1.58822705823722,4.88769531247902));
#3537=CARTESIAN_POINT('Ctrl Pts',(1.8045977690979,-1.73793406786513,4.67143479701259));
#3538=CARTESIAN_POINT('Ctrl Pts',(1.63722753567886,-1.89188688795684,4.30939601525252));
#3539=CARTESIAN_POINT('Ctrl Pts',(1.5885955233965,-1.93189082089362,4.18228427785571));
#3540=CARTESIAN_POINT('Ctrl Pts',(1.52048542524434,-1.98596995629194,3.91966465750307));
#3541=CARTESIAN_POINT('Ctrl Pts',(1.50123911195662,-2.00007126058529,3.78410209416443));
#3542=CARTESIAN_POINT('Ctrl Pts',(1.50123911195662,-2.00007126058529,3.64739446828387));
#3543=CARTESIAN_POINT('',(2.50080065552765,2.03424716928038E-17,1.64732320769858));
#3544=CARTESIAN_POINT('Ctrl Pts',(1.50123911195662,-2.00007126058529,3.64739446828387));
#3545=CARTESIAN_POINT('Ctrl Pts',(1.50123911195662,-2.00007126058529,3.51068684240331));
#3546=CARTESIAN_POINT('Ctrl Pts',(1.52048542524434,-1.98596995629194,3.37512427906467));
#3547=CARTESIAN_POINT('Ctrl Pts',(1.5885955233965,-1.93189082089362,3.11250465871203));
#3548=CARTESIAN_POINT('Ctrl Pts',(1.63722753567886,-1.89188688795684,2.98539292131522));
#3549=CARTESIAN_POINT('Ctrl Pts',(1.8045977690979,-1.73793406786513,2.62335413955515));
#3550=CARTESIAN_POINT('Ctrl Pts',(1.94320134506485,-1.58822705823722,2.40709362408872));
#3551=CARTESIAN_POINT('Ctrl Pts',(2.1780735274369,-1.24570166067483,2.06456822652633));
#3552=CARTESIAN_POINT('Ctrl Pts',(2.29374488883448,-1.02924237889175,1.9119099622171));
#3553=CARTESIAN_POINT('Ctrl Pts',(2.45559485322071,-0.53912865159993,1.70302130041923));
#3554=CARTESIAN_POINT('Ctrl Pts',(2.50080065552765,-0.264926868087175,1.64732320769858));
#3555=CARTESIAN_POINT('Ctrl Pts',(2.50080065552765,-1.38777878078145E-16,
1.64732320769858));
#3556=CARTESIAN_POINT('',(2.50080065552765,-3.06259751809754E-16,0.219135539308519));
#3557=CARTESIAN_POINT('',(2.50080065552765,-3.06259751809754E-16,7.74376865817678));
#3558=CARTESIAN_POINT('Origin',(0.,0.,0.219135539308519));
#3559=CARTESIAN_POINT('Ctrl Pts',(2.50080065552765,2.77555756156289E-16,
1.64732320769858));
#3560=CARTESIAN_POINT('Ctrl Pts',(2.50080065552765,0.264926868087175,1.64732320769858));
#3561=CARTESIAN_POINT('Ctrl Pts',(2.45559485322071,0.539128651599931,1.70302130041923));
#3562=CARTESIAN_POINT('Ctrl Pts',(2.29374488883448,1.02924237889175,1.9119099622171));
#3563=CARTESIAN_POINT('Ctrl Pts',(2.1780735274369,1.24570166067483,2.06456822652633));
#3564=CARTESIAN_POINT('Ctrl Pts',(1.96890768376227,1.55073826840574,2.36960483425724));
#3565=CARTESIAN_POINT('Ctrl Pts',(1.86390655010446,1.67272836391103,2.53212241175439));
#3566=CARTESIAN_POINT('Ctrl Pts',(1.76862293784399,1.76804321848184,2.71234996399565));
#3567=CARTESIAN_POINT('Ctrl Pts',(1.76857489488806,1.76809127588459,4.58234809684521));
#3568=CARTESIAN_POINT('Ctrl Pts',(1.863870991968,1.67276911284068,4.76261188718499));
#3569=CARTESIAN_POINT('Ctrl Pts',(1.96889195571996,1.55076120536613,4.92516116535011));
#3570=CARTESIAN_POINT('Ctrl Pts',(2.1780735274369,1.24570166067483,5.23022071004141));
#3571=CARTESIAN_POINT('Ctrl Pts',(2.29374488883448,1.02924237889175,5.38287897435064));
#3572=CARTESIAN_POINT('Ctrl Pts',(2.45559485322071,0.539128651599931,5.59176763614851));
#3573=CARTESIAN_POINT('Ctrl Pts',(2.50080065552765,0.264926868087175,5.64746572886916));
#3574=CARTESIAN_POINT('Ctrl Pts',(2.50080065552765,4.85722573273506E-16,
5.64746572886916));
#3575=CARTESIAN_POINT('Origin',(0.,0.,3.64739446828387));
#3576=CARTESIAN_POINT('',(6.65286936961679,-2.00007126058529,3.64739446828387));
#3577=CARTESIAN_POINT('',(0.,-2.00007126058529,3.64739446828387));
#3578=CARTESIAN_POINT('',(6.94701057265674,-5.29465121630953E-16,1.64732320769858));
#3579=CARTESIAN_POINT('Ctrl Pts',(6.94701057265674,-4.16333634234434E-16,
1.64732320769858));
#3580=CARTESIAN_POINT('Ctrl Pts',(6.94701057265674,-0.252651925025299,1.64732320769858));
#3581=CARTESIAN_POINT('Ctrl Pts',(6.93185967642424,-0.521185316397251,1.69810717591289));
#3582=CARTESIAN_POINT('Ctrl Pts',(6.87713670157391,-1.01355981516441,1.9026734267681));
#3583=CARTESIAN_POINT('Ctrl Pts',(6.83828274623297,-1.23751236388673,2.05637892973823));
#3584=CARTESIAN_POINT('Ctrl Pts',(6.76476847582112,-1.59105989763386,2.40992646348536));
#3585=CARTESIAN_POINT('Ctrl Pts',(6.7251858181423,-1.74473098673958,2.63386086947574));
#3586=CARTESIAN_POINT('Ctrl Pts',(6.66877424579284,-1.94927190878348,3.12616984589068));
#3587=CARTESIAN_POINT('Ctrl Pts',(6.65286936961679,-2.00007126058529,3.39467913557324));
#3588=CARTESIAN_POINT('Ctrl Pts',(6.65286936961679,-2.00007126058529,3.64739446828387));
#3589=CARTESIAN_POINT('',(6.94701057265674,-1.47825956916056E-16,5.64746572886916));
#3590=CARTESIAN_POINT('Ctrl Pts',(6.94701057265674,6.59194920871187E-16,
5.64746572886916));
#3591=CARTESIAN_POINT('Ctrl Pts',(6.94701057265674,0.252651925025299,5.64746572886916));
#3592=CARTESIAN_POINT('Ctrl Pts',(6.93185967642424,0.521185316397251,5.59668176065485));
#3593=CARTESIAN_POINT('Ctrl Pts',(6.87713670157391,1.01355981516441,5.39211550979964));
#3594=CARTESIAN_POINT('Ctrl Pts',(6.83828274623297,1.23751236388673,5.23841000682951));
#3595=CARTESIAN_POINT('Ctrl Pts',(6.76476847582112,1.59105989763386,4.88486247308238));
#3596=CARTESIAN_POINT('Ctrl Pts',(6.7251858181423,1.74473098673958,4.660928067092));
#3597=CARTESIAN_POINT('Ctrl Pts',(6.66877424579284,1.94927190878348,4.16861909067706));
#3598=CARTESIAN_POINT('Ctrl Pts',(6.65286936961679,2.00007126058529,3.9001098009945));
#3599=CARTESIAN_POINT('Ctrl Pts',(6.65286936961679,2.00007126058529,3.39467913557324));
#3600=CARTESIAN_POINT('Ctrl Pts',(6.66877424579284,1.94927190878348,3.12616984589068));
#3601=CARTESIAN_POINT('Ctrl Pts',(6.7251858181423,1.74473098673958,2.63386086947574));
#3602=CARTESIAN_POINT('Ctrl Pts',(6.76476847582112,1.59105989763386,2.40992646348536));
#3603=CARTESIAN_POINT('Ctrl Pts',(6.83828274623297,1.23751236388673,2.05637892973823));
#3604=CARTESIAN_POINT('Ctrl Pts',(6.87713670157391,1.01355981516441,1.9026734267681));
#3605=CARTESIAN_POINT('Ctrl Pts',(6.93185967642424,0.52118531639725,1.69810717591289));
#3606=CARTESIAN_POINT('Ctrl Pts',(6.94701057265674,0.252651925025298,1.64732320769858));
#3607=CARTESIAN_POINT('Ctrl Pts',(6.94701057265674,-4.16333634234434E-16,
1.64732320769858));
#3608=CARTESIAN_POINT('Ctrl Pts',(6.65286936961679,-2.00007126058529,3.64739446828387));
#3609=CARTESIAN_POINT('Ctrl Pts',(6.65286936961679,-2.00007126058529,3.9001098009945));
#3610=CARTESIAN_POINT('Ctrl Pts',(6.66877424579284,-1.94927190878348,4.16861909067706));
#3611=CARTESIAN_POINT('Ctrl Pts',(6.7251858181423,-1.74473098673957,4.660928067092));
#3612=CARTESIAN_POINT('Ctrl Pts',(6.76476847582112,-1.59105989763386,4.88486247308238));
#3613=CARTESIAN_POINT('Ctrl Pts',(6.83828274623297,-1.23751236388673,5.23841000682951));
#3614=CARTESIAN_POINT('Ctrl Pts',(6.87713670157391,-1.01355981516441,5.39211550979964));
#3615=CARTESIAN_POINT('Ctrl Pts',(6.93185967642424,-0.52118531639725,5.59668176065485));
#3616=CARTESIAN_POINT('Ctrl Pts',(6.94701057265674,-0.252651925025297,5.64746572886916));
#3617=CARTESIAN_POINT('Ctrl Pts',(6.94701057265674,8.32667268468867E-16,
5.64746572886916));
#3618=CARTESIAN_POINT('Origin',(4.58300560234995,1.11126133386797,7.30323111171487));
#3619=CARTESIAN_POINT('',(4.5963952096795,1.23456935960356,7.30323111171487));
#3620=CARTESIAN_POINT('',(4.5963952096795,1.23456935960356,14.3002311117149));
#3621=CARTESIAN_POINT('',(4.5963952096795,1.23456935960356,7.30323111171487));
#3622=CARTESIAN_POINT('',(4.5578337263362,1.23271308335391,7.30323111171487));
#3623=CARTESIAN_POINT('Origin',(4.58300560234995,1.11126133386797,7.30323111171487));
#3624=CARTESIAN_POINT('',(4.5578337263362,1.23271308335391,14.3002311117149));
#3625=CARTESIAN_POINT('',(4.5578337263362,1.23271308335391,7.30323111171487));
#3626=CARTESIAN_POINT('Origin',(4.58300560234995,1.11126133386797,14.3002311117149));
#3627=CARTESIAN_POINT('Origin',(4.69562204444668,2.09062562955478,14.3002311117149));
#3628=CARTESIAN_POINT('',(3.99305254500011,2.58969917173881,14.3002311117149));
#3629=CARTESIAN_POINT('Origin',(0.,0.,14.3002311117149));
#3630=CARTESIAN_POINT('',(3.96587039417894,2.562284496182,14.3002311117149));
#3631=CARTESIAN_POINT('Origin',(4.42403620092708,1.96970782149614,14.3002311117149));
#3632=CARTESIAN_POINT('Origin',(3.89245742766355,2.66225792836605,14.3002311117149));
#3633=CARTESIAN_POINT('Origin',(4.42403620092708,1.96970782149614,7.30323111171487));
#3634=CARTESIAN_POINT('',(3.96587039417894,2.562284496182,7.30323111171487));
#3635=CARTESIAN_POINT('Origin',(4.42403620092708,1.96970782149614,7.30323111171487));
#3636=CARTESIAN_POINT('',(3.96587039417894,2.562284496182,7.30323111171487));
#3637=CARTESIAN_POINT('Origin',(3.89245742766355,2.66225792836605,7.30323111171487));
#3638=CARTESIAN_POINT('',(3.99305254500011,2.58969917173881,7.30323111171487));
#3639=CARTESIAN_POINT('',(3.99305254500011,2.58969917173881,7.30323111171487));
#3640=CARTESIAN_POINT('Origin',(3.89245742766355,2.66225792836605,7.30323111171487));
#3641=CARTESIAN_POINT('Origin',(3.73479324586,2.87926405770635,7.30323111171487));
#3642=CARTESIAN_POINT('',(3.69687136836352,2.99735758844529,7.30323111171487));
#3643=CARTESIAN_POINT('',(3.69687136836352,2.99735758844529,14.3002311117149));
#3644=CARTESIAN_POINT('',(3.69687136836352,2.99735758844529,7.30323111171487));
#3645=CARTESIAN_POINT('',(3.6623987159857,2.97997742742222,7.30323111171487));
#3646=CARTESIAN_POINT('Origin',(3.73479324586,2.87926405770635,7.30323111171487));
#3647=CARTESIAN_POINT('',(3.6623987159857,2.97997742742222,14.3002311117149));
#3648=CARTESIAN_POINT('',(3.6623987159857,2.97997742742222,7.30323111171487));
#3649=CARTESIAN_POINT('Origin',(3.73479324586,2.87926405770635,14.3002311117149));
#3650=CARTESIAN_POINT('Origin',(3.43933013901738,3.81976309502194,14.3002311117149));
#3651=CARTESIAN_POINT('',(2.59450946692386,3.98992870278142,14.3002311117149));
#3652=CARTESIAN_POINT('Origin',(0.,0.,14.3002311117149));
#3653=CARTESIAN_POINT('',(2.5808278896192,3.95382817367717,14.3002311117149));
#3654=CARTESIAN_POINT('Origin',(3.24040582864787,3.59883526642179,14.3002311117149));
#3655=CARTESIAN_POINT('Origin',(2.4730989493237,4.01529870497514,14.3002311117149));
#3656=CARTESIAN_POINT('Origin',(3.24040582864787,3.59883526642179,7.30323111171487));
#3657=CARTESIAN_POINT('',(2.5808278896192,3.95382817367717,7.30323111171487));
#3658=CARTESIAN_POINT('Origin',(3.24040582864787,3.59883526642179,7.30323111171487));
#3659=CARTESIAN_POINT('',(2.5808278896192,3.95382817367717,7.30323111171487));
#3660=CARTESIAN_POINT('Origin',(2.4730989493237,4.01529870497514,7.30323111171487));
#3661=CARTESIAN_POINT('',(2.59450946692386,3.98992870278142,7.30323111171487));
#3662=CARTESIAN_POINT('',(2.59450946692386,3.98992870278142,7.30323111171487));
#3663=CARTESIAN_POINT('Origin',(2.4730989493237,4.01529870497514,7.30323111171487));
#3664=CARTESIAN_POINT('Origin',(2.24080120762938,4.1494158686745,7.30323111171487));
#3665=CARTESIAN_POINT('',(2.15812488243547,4.241875460106,7.30323111171487));
#3666=CARTESIAN_POINT('',(2.15812488243547,4.241875460106,14.3002311117149));
#3667=CARTESIAN_POINT('',(2.15812488243547,4.241875460106,7.30323111171487));
#3668=CARTESIAN_POINT('',(2.13370169579345,4.2119766020442,7.30323111171487));
#3669=CARTESIAN_POINT('Origin',(2.24080120762938,4.1494158686745,7.30323111171487));
#3670=CARTESIAN_POINT('',(2.13370169579345,4.2119766020442,14.3002311117149));
#3671=CARTESIAN_POINT('',(2.13370169579345,4.2119766020442,7.30323111171487));
#3672=CARTESIAN_POINT('Origin',(2.24080120762938,4.1494158686745,14.3002311117149));
#3673=CARTESIAN_POINT('Origin',(1.58834680721857,4.88842881990149,14.3002311117149));
#3674=CARTESIAN_POINT('',(0.74735213163792,4.7002633137488,14.3002311117149));
#3675=CARTESIAN_POINT('Origin',(0.,0.,14.3002311117149));
#3676=CARTESIAN_POINT('',(0.749536796858992,4.66171904054223,14.3002311117149));
#3677=CARTESIAN_POINT('Origin',(1.49647985043267,4.60569139939112,14.3002311117149));
#3678=CARTESIAN_POINT('Origin',(0.62611919524716,4.67405785765047,14.3002311117149));
#3679=CARTESIAN_POINT('Origin',(1.49647985043267,4.60569139939112,7.30323111171487));
#3680=CARTESIAN_POINT('',(0.749536796858992,4.66171904054223,7.30323111171487));
#3681=CARTESIAN_POINT('Origin',(1.49647985043267,4.60569139939112,7.30323111171487));
#3682=CARTESIAN_POINT('',(0.749536796858992,4.66171904054223,7.30323111171487));
#3683=CARTESIAN_POINT('Origin',(0.62611919524716,4.67405785765047,7.30323111171487));
#3684=CARTESIAN_POINT('',(0.74735213163792,4.7002633137488,7.30323111171487));
#3685=CARTESIAN_POINT('',(0.74735213163792,4.7002633137488,7.30323111171487));
#3686=CARTESIAN_POINT('Origin',(0.62611919524716,4.67405785765047,7.30323111171487));
#3687=CARTESIAN_POINT('Origin',(0.359354283559748,4.70209597968909,7.30323111171487));
#3688=CARTESIAN_POINT('',(0.246218998385265,4.75293452848561,7.30323111171487));
#3689=CARTESIAN_POINT('',(0.246218998385265,4.75293452848561,14.3002311117149));
#3690=CARTESIAN_POINT('',(0.246218998385265,4.75293452848561,7.30323111171487));
#3691=CARTESIAN_POINT('',(0.236068268327149,4.71568675756656,7.30323111171487));
#3692=CARTESIAN_POINT('Origin',(0.359354283559748,4.70209597968909,7.30323111171487));
#3693=CARTESIAN_POINT('',(0.236068268327149,4.71568675756656,14.3002311117149));
#3694=CARTESIAN_POINT('',(0.236068268327149,4.71568675756656,7.30323111171487));
#3695=CARTESIAN_POINT('Origin',(0.359354283559748,4.70209597968909,14.3002311117149));
#3696=CARTESIAN_POINT('Origin',(-0.537276117226072,5.11184079183843,14.3002311117149));
#3697=CARTESIAN_POINT('',(-1.22902917668919,4.59787969721732,14.3002311117149));
#3698=CARTESIAN_POINT('Origin',(0.,0.,14.3002311117149));
#3699=CARTESIAN_POINT('',(-1.21135601740617,4.5635563349096,14.3002311117149));
#3700=CARTESIAN_POINT('Origin',(-0.506201089014987,4.81618164801291,14.3002311117149));
#3701=CARTESIAN_POINT('Origin',(-1.32912225580194,4.52462994425545,14.3002311117149));
#3702=CARTESIAN_POINT('Origin',(-0.506201089014987,4.81618164801291,7.30323111171487));
#3703=CARTESIAN_POINT('',(-1.21135601740617,4.5635563349096,7.30323111171487));
#3704=CARTESIAN_POINT('Origin',(-0.506201089014987,4.81618164801291,7.30323111171487));
#3705=CARTESIAN_POINT('',(-1.21135601740617,4.5635563349096,7.30323111171487));
#3706=CARTESIAN_POINT('Origin',(-1.32912225580194,4.52462994425545,7.30323111171487));
#3707=CARTESIAN_POINT('',(-1.22902917668919,4.59787969721732,7.30323111171487));
#3708=CARTESIAN_POINT('',(-1.22902917668919,4.59787969721732,7.30323111171487));
#3709=CARTESIAN_POINT('Origin',(-1.32912225580194,4.52462994425545,7.30323111171487));
#3710=CARTESIAN_POINT('Origin',(-1.58422826076854,4.44174097861451,7.30323111171487));
#3711=CARTESIAN_POINT('',(-1.70826038731513,4.44216803783541,7.30323111171487));
#3712=CARTESIAN_POINT('',(-1.70826038731513,4.44216803783541,14.3002311117149));
#3713=CARTESIAN_POINT('',(-1.70826038731513,4.44216803783541,7.30323111171487));
#3714=CARTESIAN_POINT('',(-1.70238350734581,4.4040118320364,7.30323111171487));
#3715=CARTESIAN_POINT('Origin',(-1.58422826076854,4.44174097861451,7.30323111171487));
#3716=CARTESIAN_POINT('',(-1.70238350734581,4.4040118320364,14.3002311117149));
#3717=CARTESIAN_POINT('',(-1.70238350734581,4.4040118320364,7.30323111171487));
#3718=CARTESIAN_POINT('Origin',(-1.58422826076854,4.44174097861451,14.3002311117149));
#3719=CARTESIAN_POINT('Origin',(-2.56999912000204,4.45136905125082,14.3002311117149));
#3720=CARTESIAN_POINT('',(-2.99290017498718,3.70048091061125,14.3002311117149));
#3721=CARTESIAN_POINT('Origin',(0.,0.,14.3002311117149));
#3722=CARTESIAN_POINT('',(-2.96279437143787,3.67631328036332,14.3002311117149));
#3723=CARTESIAN_POINT('Origin',(-2.42135526147943,4.19391033605658,14.3002311117149));
#3724=CARTESIAN_POINT('Origin',(-3.05454639412625,3.59285240852604,14.3002311117149));
#3725=CARTESIAN_POINT('Origin',(-2.42135526147943,4.19391033605658,7.30323111171487));
#3726=CARTESIAN_POINT('',(-2.96279437143787,3.67631328036332,7.30323111171487));
#3727=CARTESIAN_POINT('Origin',(-2.42135526147943,4.19391033605658,7.30323111171487));
#3728=CARTESIAN_POINT('',(-2.96279437143787,3.67631328036332,7.30323111171487));
#3729=CARTESIAN_POINT('Origin',(-3.05454639412625,3.59285240852604,7.30323111171487));
#3730=CARTESIAN_POINT('',(-2.99290017498718,3.70048091061125,7.30323111171487));
#3731=CARTESIAN_POINT('',(-2.99290017498718,3.70048091061125,7.30323111171487));
#3732=CARTESIAN_POINT('Origin',(-3.05454639412625,3.59285240852604,7.30323111171487));
#3733=CARTESIAN_POINT('Origin',(-3.25388334654802,3.41336861038748,7.30323111171487));
#3734=CARTESIAN_POINT('',(-3.36736603299031,3.36331033761377,7.30323111171487));
#3735=CARTESIAN_POINT('',(-3.36736603299031,3.36331033761377,14.3002311117149));
#3736=CARTESIAN_POINT('',(-3.36736603299031,3.36331033761377,7.30323111171487));
#3737=CARTESIAN_POINT('',(-3.34647770893003,3.33084325155569,7.30323111171487));
#3738=CARTESIAN_POINT('Origin',(-3.25388334654802,3.41336861038748,7.30323111171487));
#3739=CARTESIAN_POINT('',(-3.34647770893003,3.33084325155569,14.3002311117149));
#3740=CARTESIAN_POINT('',(-3.34647770893003,3.33084325155569,7.30323111171487));
#3741=CARTESIAN_POINT('Origin',(-3.25388334654802,3.41336861038748,14.3002311117149));
#3742=CARTESIAN_POINT('Origin',(-4.15834592722061,3.02121516228366,14.3002311117149));
#3743=CARTESIAN_POINT('',(-4.23927154338538,2.1632353567468,14.3002311117149));
#3744=CARTESIAN_POINT('Origin',(0.,0.,14.3002311117149));
#3745=CARTESIAN_POINT('',(-4.20193866250609,2.15340226138457,14.3002311117149));
#3746=CARTESIAN_POINT('Origin',(-3.9178351119121,2.84647382651678,14.3002311117149));
#3747=CARTESIAN_POINT('Origin',(-4.25181171122331,2.03983805132304,14.3002311117149));
#3748=CARTESIAN_POINT('Origin',(-3.9178351119121,2.84647382651678,7.30323111171487));
#3749=CARTESIAN_POINT('',(-4.20193866250609,2.15340226138457,7.30323111171487));
#3750=CARTESIAN_POINT('Origin',(-3.9178351119121,2.84647382651678,7.30323111171487));
#3751=CARTESIAN_POINT('',(-4.20193866250609,2.15340226138457,7.30323111171487));
#3752=CARTESIAN_POINT('Origin',(-4.25181171122331,2.03983805132304,7.30323111171487));
#3753=CARTESIAN_POINT('',(-4.23927154338538,2.1632353567468,7.30323111171487));
#3754=CARTESIAN_POINT('',(-4.23927154338538,2.1632353567468,7.30323111171487));
#3755=CARTESIAN_POINT('Origin',(-4.25181171122331,2.03983805132304,7.30323111171487));
#3756=CARTESIAN_POINT('Origin',(-4.36091244110716,1.79479379994412,7.30323111171487));
#3757=CARTESIAN_POINT('',(-4.44422350000145,1.70290572530351,7.30323111171487));
#3758=CARTESIAN_POINT('',(-4.44422350000145,1.70290572530351,14.3002311117149));
#3759=CARTESIAN_POINT('',(-4.44422350000145,1.70290572530351,7.30323111171487));
#3760=CARTESIAN_POINT('',(-4.41193551284469,1.68174161312001,7.30323111171487));
#3761=CARTESIAN_POINT('Origin',(-4.36091244110716,1.79479379994412,7.30323111171487));
#3762=CARTESIAN_POINT('',(-4.41193551284469,1.68174161312001,14.3002311117149));
#3763=CARTESIAN_POINT('',(-4.41193551284469,1.68174161312001,7.30323111171487));
#3764=CARTESIAN_POINT('Origin',(-4.36091244110716,1.79479379994412,14.3002311117149));
#3765=CARTESIAN_POINT('Origin',(-5.02767694623596,1.06866572487955,14.3002311117149));
#3766=CARTESIAN_POINT('',(-4.75263434935933,0.251946757324573,14.3002311117149));
#3767=CARTESIAN_POINT('Origin',(0.,0.,14.3002311117149));
#3768=CARTESIAN_POINT('',(-4.71452958541266,0.258148428367029,14.3002311117149));
#3769=CARTESIAN_POINT('Origin',(-4.73688567908055,1.00685613296933,14.3002311117149));
#3770=CARTESIAN_POINT('Origin',(-4.71390015695308,0.134117163699359,14.3002311117149));
#3771=CARTESIAN_POINT('Origin',(-4.73688567908055,1.00685613296933,7.30323111171487));
#3772=CARTESIAN_POINT('',(-4.71452958541266,0.258148428367029,7.30323111171487));
#3773=CARTESIAN_POINT('Origin',(-4.73688567908055,1.00685613296933,7.30323111171487));
#3774=CARTESIAN_POINT('',(-4.71452958541266,0.258148428367029,7.30323111171487));
#3775=CARTESIAN_POINT('Origin',(-4.71390015695308,0.134117163699359,7.30323111171487));
#3776=CARTESIAN_POINT('',(-4.75263434935933,0.251946757324573,7.30323111171487));
#3777=CARTESIAN_POINT('',(-4.75263434935933,0.251946757324573,7.30323111171487));
#3778=CARTESIAN_POINT('Origin',(-4.71390015695308,0.134117163699359,7.30323111171487));
#3779=CARTESIAN_POINT('Origin',(-4.71390015695308,-0.134117163699362,7.30323111171487));
#3780=CARTESIAN_POINT('',(-4.75263434935933,-0.251946757324576,7.30323111171487));
#3781=CARTESIAN_POINT('',(-4.75263434935933,-0.251946757324576,14.3002311117149));
#3782=CARTESIAN_POINT('',(-4.75263434935933,-0.251946757324576,7.30323111171487));
#3783=CARTESIAN_POINT('',(-4.71452958541266,-0.258148428367032,7.30323111171487));
#3784=CARTESIAN_POINT('Origin',(-4.71390015695308,-0.134117163699362,7.30323111171487));
#3785=CARTESIAN_POINT('',(-4.71452958541266,-0.258148428367032,14.3002311117149));
#3786=CARTESIAN_POINT('',(-4.71452958541266,-0.258148428367032,7.30323111171487));
#3787=CARTESIAN_POINT('Origin',(-4.71390015695308,-0.134117163699362,14.3002311117149));
#3788=CARTESIAN_POINT('Origin',(-5.02767694623596,-1.06866572487955,14.3002311117149));
#3789=CARTESIAN_POINT('',(-4.44422350000145,-1.70290572530351,14.3002311117149));
#3790=CARTESIAN_POINT('Origin',(0.,0.,14.3002311117149));
#3791=CARTESIAN_POINT('',(-4.41193551284469,-1.68174161312001,14.3002311117149));
#3792=CARTESIAN_POINT('Origin',(-4.73688567908055,-1.00685613296933,14.3002311117149));
#3793=CARTESIAN_POINT('Origin',(-4.36091244110716,-1.79479379994413,14.3002311117149));
#3794=CARTESIAN_POINT('Origin',(-4.73688567908055,-1.00685613296933,7.30323111171487));
#3795=CARTESIAN_POINT('',(-4.41193551284469,-1.68174161312001,7.30323111171487));
#3796=CARTESIAN_POINT('Origin',(-4.73688567908055,-1.00685613296933,7.30323111171487));
#3797=CARTESIAN_POINT('',(-4.41193551284469,-1.68174161312001,7.30323111171487));
#3798=CARTESIAN_POINT('Origin',(-4.36091244110716,-1.79479379994413,7.30323111171487));
#3799=CARTESIAN_POINT('',(-4.44422350000145,-1.70290572530351,7.30323111171487));
#3800=CARTESIAN_POINT('',(-4.44422350000145,-1.70290572530351,7.30323111171487));
#3801=CARTESIAN_POINT('Origin',(-4.36091244110716,-1.79479379994413,7.30323111171487));
#3802=CARTESIAN_POINT('Origin',(-4.25181171122331,-2.03983805132304,7.30323111171487));
#3803=CARTESIAN_POINT('',(-4.23927154338538,-2.1632353567468,7.30323111171487));
#3804=CARTESIAN_POINT('',(-4.23927154338538,-2.1632353567468,14.3002311117149));
#3805=CARTESIAN_POINT('',(-4.23927154338538,-2.1632353567468,7.30323111171487));
#3806=CARTESIAN_POINT('',(-4.20193866250609,-2.15340226138457,7.30323111171487));
#3807=CARTESIAN_POINT('Origin',(-4.25181171122331,-2.03983805132304,7.30323111171487));
#3808=CARTESIAN_POINT('',(-4.20193866250609,-2.15340226138457,14.3002311117149));
#3809=CARTESIAN_POINT('',(-4.20193866250609,-2.15340226138457,7.30323111171487));
#3810=CARTESIAN_POINT('Origin',(-4.25181171122331,-2.03983805132304,14.3002311117149));
#3811=CARTESIAN_POINT('Origin',(-4.15834592722061,-3.02121516228366,14.3002311117149));
#3812=CARTESIAN_POINT('',(-3.36736603299031,-3.36331033761377,14.3002311117149));
#3813=CARTESIAN_POINT('Origin',(0.,0.,14.3002311117149));
#3814=CARTESIAN_POINT('',(-3.34647770893003,-3.33084325155569,14.3002311117149));
#3815=CARTESIAN_POINT('Origin',(-3.91783511191209,-2.84647382651678,14.3002311117149));
#3816=CARTESIAN_POINT('Origin',(-3.25388334654802,-3.41336861038748,14.3002311117149));
#3817=CARTESIAN_POINT('Origin',(-3.91783511191209,-2.84647382651678,7.30323111171487));
#3818=CARTESIAN_POINT('',(-3.34647770893003,-3.33084325155569,7.30323111171487));
#3819=CARTESIAN_POINT('Origin',(-3.91783511191209,-2.84647382651678,7.30323111171487));
#3820=CARTESIAN_POINT('',(-3.34647770893003,-3.33084325155569,7.30323111171487));
#3821=CARTESIAN_POINT('Origin',(-3.25388334654802,-3.41336861038748,7.30323111171487));
#3822=CARTESIAN_POINT('',(-3.36736603299031,-3.36331033761377,7.30323111171487));
#3823=CARTESIAN_POINT('',(-3.36736603299031,-3.36331033761377,7.30323111171487));
#3824=CARTESIAN_POINT('Origin',(-3.25388334654802,-3.41336861038748,7.30323111171487));
#3825=CARTESIAN_POINT('Origin',(-3.05454639412625,-3.59285240852604,7.30323111171487));
#3826=CARTESIAN_POINT('',(-2.99290017498718,-3.70048091061125,7.30323111171487));
#3827=CARTESIAN_POINT('',(-2.99290017498718,-3.70048091061125,14.3002311117149));
#3828=CARTESIAN_POINT('',(-2.99290017498718,-3.70048091061125,7.30323111171487));
#3829=CARTESIAN_POINT('',(-2.96279437143787,-3.67631328036332,7.30323111171487));
#3830=CARTESIAN_POINT('Origin',(-3.05454639412625,-3.59285240852604,7.30323111171487));
#3831=CARTESIAN_POINT('',(-2.96279437143787,-3.67631328036332,14.3002311117149));
#3832=CARTESIAN_POINT('',(-2.96279437143787,-3.67631328036332,7.30323111171487));
#3833=CARTESIAN_POINT('Origin',(-3.05454639412625,-3.59285240852604,14.3002311117149));
#3834=CARTESIAN_POINT('Origin',(-2.56999912000203,-4.45136905125083,14.3002311117149));
#3835=CARTESIAN_POINT('',(-1.70826038731512,-4.44216803783542,14.3002311117149));
#3836=CARTESIAN_POINT('Origin',(0.,0.,14.3002311117149));
#3837=CARTESIAN_POINT('',(-1.7023835073458,-4.4040118320364,14.3002311117149));
#3838=CARTESIAN_POINT('Origin',(-2.42135526147942,-4.19391033605659,14.3002311117149));
#3839=CARTESIAN_POINT('Origin',(-1.58422826076853,-4.44174097861451,14.3002311117149));
#3840=CARTESIAN_POINT('Origin',(-2.42135526147942,-4.19391033605659,7.30323111171487));
#3841=CARTESIAN_POINT('',(-1.7023835073458,-4.4040118320364,7.30323111171487));
#3842=CARTESIAN_POINT('Origin',(-2.42135526147942,-4.19391033605659,7.30323111171487));
#3843=CARTESIAN_POINT('',(-1.7023835073458,-4.4040118320364,7.30323111171487));
#3844=CARTESIAN_POINT('Origin',(-1.58422826076853,-4.44174097861451,7.30323111171487));
#3845=CARTESIAN_POINT('',(-1.70826038731512,-4.44216803783542,7.30323111171487));
#3846=CARTESIAN_POINT('',(-1.70826038731512,-4.44216803783542,7.30323111171487));
#3847=CARTESIAN_POINT('Origin',(-1.58422826076853,-4.44174097861451,7.30323111171487));
#3848=CARTESIAN_POINT('Origin',(-1.32912225580193,-4.52462994425545,7.30323111171487));
#3849=CARTESIAN_POINT('',(-1.22902917668918,-4.59787969721732,7.30323111171487));
#3850=CARTESIAN_POINT('',(-1.22902917668918,-4.59787969721732,14.3002311117149));
#3851=CARTESIAN_POINT('',(-1.22902917668918,-4.59787969721732,7.30323111171487));
#3852=CARTESIAN_POINT('',(-1.21135601740617,-4.5635563349096,7.30323111171487));
#3853=CARTESIAN_POINT('Origin',(-1.32912225580193,-4.52462994425545,7.30323111171487));
#3854=CARTESIAN_POINT('',(-1.21135601740617,-4.5635563349096,14.3002311117149));
#3855=CARTESIAN_POINT('',(-1.21135601740617,-4.5635563349096,7.30323111171487));
#3856=CARTESIAN_POINT('Origin',(-1.32912225580193,-4.52462994425545,14.3002311117149));
#3857=CARTESIAN_POINT('Origin',(-0.537276117226068,-5.11184079183843,14.3002311117149));
#3858=CARTESIAN_POINT('',(0.246218998385269,-4.75293452848561,14.3002311117149));
#3859=CARTESIAN_POINT('Origin',(0.,0.,14.3002311117149));
#3860=CARTESIAN_POINT('',(0.236068268327154,-4.71568675756656,14.3002311117149));
#3861=CARTESIAN_POINT('Origin',(-0.506201089014981,-4.81618164801291,14.3002311117149));
#3862=CARTESIAN_POINT('Origin',(0.359354283559752,-4.70209597968909,14.3002311117149));
#3863=CARTESIAN_POINT('Origin',(-0.506201089014981,-4.81618164801291,7.30323111171487));
#3864=CARTESIAN_POINT('',(0.236068268327154,-4.71568675756656,7.30323111171487));
#3865=CARTESIAN_POINT('Origin',(-0.506201089014981,-4.81618164801291,7.30323111171487));
#3866=CARTESIAN_POINT('',(0.236068268327154,-4.71568675756656,7.30323111171487));
#3867=CARTESIAN_POINT('Origin',(0.359354283559752,-4.70209597968909,7.30323111171487));
#3868=CARTESIAN_POINT('',(0.246218998385269,-4.75293452848561,7.30323111171487));
#3869=CARTESIAN_POINT('',(0.246218998385269,-4.75293452848561,7.30323111171487));
#3870=CARTESIAN_POINT('Origin',(0.359354283559752,-4.70209597968909,7.30323111171487));
#3871=CARTESIAN_POINT('Origin',(0.626119195247162,-4.67405785765047,7.30323111171487));
#3872=CARTESIAN_POINT('',(0.747352131637922,-4.7002633137488,7.30323111171487));
#3873=CARTESIAN_POINT('',(0.747352131637922,-4.7002633137488,14.3002311117149));
#3874=CARTESIAN_POINT('',(0.747352131637922,-4.7002633137488,7.30323111171487));
#3875=CARTESIAN_POINT('',(0.749536796858993,-4.66171904054223,7.30323111171487));
#3876=CARTESIAN_POINT('Origin',(0.626119195247162,-4.67405785765047,7.30323111171487));
#3877=CARTESIAN_POINT('',(0.749536796858993,-4.66171904054223,14.3002311117149));
#3878=CARTESIAN_POINT('',(0.749536796858993,-4.66171904054223,7.30323111171487));
#3879=CARTESIAN_POINT('Origin',(0.626119195247162,-4.67405785765047,14.3002311117149));
#3880=CARTESIAN_POINT('Origin',(1.58834680721858,-4.88842881990149,14.3002311117149));
#3881=CARTESIAN_POINT('',(2.15812488243547,-4.24187546010599,14.3002311117149));
#3882=CARTESIAN_POINT('Origin',(0.,0.,14.3002311117149));
#3883=CARTESIAN_POINT('',(2.13370169579346,-4.2119766020442,14.3002311117149));
#3884=CARTESIAN_POINT('Origin',(1.49647985043267,-4.60569139939112,14.3002311117149));
#3885=CARTESIAN_POINT('Origin',(2.24080120762938,-4.1494158686745,14.3002311117149));
#3886=CARTESIAN_POINT('Origin',(1.49647985043267,-4.60569139939112,7.30323111171487));
#3887=CARTESIAN_POINT('',(2.13370169579346,-4.2119766020442,7.30323111171487));
#3888=CARTESIAN_POINT('Origin',(1.49647985043267,-4.60569139939112,7.30323111171487));
#3889=CARTESIAN_POINT('',(2.13370169579346,-4.2119766020442,7.30323111171487));
#3890=CARTESIAN_POINT('Origin',(2.24080120762938,-4.1494158686745,7.30323111171487));
#3891=CARTESIAN_POINT('',(2.15812488243547,-4.24187546010599,7.30323111171487));
#3892=CARTESIAN_POINT('',(2.15812488243547,-4.24187546010599,7.30323111171487));
#3893=CARTESIAN_POINT('Origin',(2.24080120762938,-4.1494158686745,7.30323111171487));
#3894=CARTESIAN_POINT('Origin',(2.4730989493237,-4.01529870497514,7.30323111171487));
#3895=CARTESIAN_POINT('',(2.59450946692386,-3.98992870278142,7.30323111171487));
#3896=CARTESIAN_POINT('',(2.59450946692386,-3.98992870278142,14.3002311117149));
#3897=CARTESIAN_POINT('',(2.59450946692386,-3.98992870278142,7.30323111171487));
#3898=CARTESIAN_POINT('',(2.58082788961921,-3.95382817367717,7.30323111171487));
#3899=CARTESIAN_POINT('Origin',(2.4730989493237,-4.01529870497514,7.30323111171487));
#3900=CARTESIAN_POINT('',(2.58082788961921,-3.95382817367717,14.3002311117149));
#3901=CARTESIAN_POINT('',(2.58082788961921,-3.95382817367717,7.30323111171487));
#3902=CARTESIAN_POINT('Origin',(2.4730989493237,-4.01529870497514,14.3002311117149));
#3903=CARTESIAN_POINT('Origin',(3.43933013901739,-3.81976309502194,14.3002311117149));
#3904=CARTESIAN_POINT('',(3.69687136836353,-2.99735758844529,14.3002311117149));
#3905=CARTESIAN_POINT('Origin',(0.,0.,14.3002311117149));
#3906=CARTESIAN_POINT('',(3.6623987159857,-2.97997742742222,14.3002311117149));
#3907=CARTESIAN_POINT('Origin',(3.24040582864788,-3.59883526642179,14.3002311117149));
#3908=CARTESIAN_POINT('Origin',(3.73479324586,-2.87926405770635,14.3002311117149));
#3909=CARTESIAN_POINT('Origin',(3.24040582864788,-3.59883526642179,7.30323111171487));
#3910=CARTESIAN_POINT('',(3.6623987159857,-2.97997742742222,7.30323111171487));
#3911=CARTESIAN_POINT('Origin',(3.24040582864788,-3.59883526642179,7.30323111171487));
#3912=CARTESIAN_POINT('',(3.6623987159857,-2.97997742742222,7.30323111171487));
#3913=CARTESIAN_POINT('Origin',(3.73479324586,-2.87926405770635,7.30323111171487));
#3914=CARTESIAN_POINT('',(3.69687136836353,-2.99735758844529,7.30323111171487));
#3915=CARTESIAN_POINT('',(3.69687136836353,-2.99735758844529,7.30323111171487));
#3916=CARTESIAN_POINT('Origin',(3.73479324586,-2.87926405770635,7.30323111171487));
#3917=CARTESIAN_POINT('Origin',(3.89245742766356,-2.66225792836605,7.30323111171487));
#3918=CARTESIAN_POINT('',(3.99305254500012,-2.58969917173881,7.30323111171487));
#3919=CARTESIAN_POINT('',(3.99305254500012,-2.58969917173881,14.3002311117149));
#3920=CARTESIAN_POINT('',(3.99305254500012,-2.58969917173881,7.30323111171487));
#3921=CARTESIAN_POINT('',(3.96587039417894,-2.562284496182,7.30323111171487));
#3922=CARTESIAN_POINT('Origin',(3.89245742766356,-2.66225792836605,7.30323111171487));
#3923=CARTESIAN_POINT('',(3.96587039417894,-2.562284496182,14.3002311117149));
#3924=CARTESIAN_POINT('',(3.96587039417894,-2.562284496182,7.30323111171487));
#3925=CARTESIAN_POINT('Origin',(3.89245742766356,-2.66225792836605,14.3002311117149));
#3926=CARTESIAN_POINT('Origin',(4.69562204444668,-2.09062562955477,14.3002311117149));
#3927=CARTESIAN_POINT('',(4.5963952096795,-1.23456935960355,14.3002311117149));
#3928=CARTESIAN_POINT('Origin',(0.,0.,14.3002311117149));
#3929=CARTESIAN_POINT('',(4.5578337263362,-1.23271308335391,14.3002311117149));
#3930=CARTESIAN_POINT('Origin',(4.42403620092708,-1.96970782149613,14.3002311117149));
#3931=CARTESIAN_POINT('Origin',(4.58300560234995,-1.11126133386797,14.3002311117149));
#3932=CARTESIAN_POINT('Origin',(4.42403620092708,-1.96970782149613,7.30323111171487));
#3933=CARTESIAN_POINT('',(4.5578337263362,-1.23271308335391,7.30323111171487));
#3934=CARTESIAN_POINT('Origin',(4.42403620092708,-1.96970782149613,7.30323111171487));
#3935=CARTESIAN_POINT('',(4.5578337263362,-1.23271308335391,7.30323111171487));
#3936=CARTESIAN_POINT('Origin',(4.58300560234995,-1.11126133386797,7.30323111171487));
#3937=CARTESIAN_POINT('',(4.5963952096795,-1.23456935960355,7.30323111171487));
#3938=CARTESIAN_POINT('',(4.5963952096795,-1.23456935960355,7.30323111171487));
#3939=CARTESIAN_POINT('Origin',(4.58300560234995,-1.11126133386797,7.30323111171487));
#3940=CARTESIAN_POINT('Origin',(0.,0.,10.8017566198263));
#3941=CARTESIAN_POINT('',(4.70116056230231,-0.741687127224166,14.3002311117149));
#3942=CARTESIAN_POINT('',(4.75930776765241,-5.82847102381266E-16,14.3002311117149));
#3943=CARTESIAN_POINT('Origin',(0.,0.,14.3002311117149));
#3944=CARTESIAN_POINT('',(4.75930776765241,-5.82847102381266E-16,14.3002821279377));
#3945=CARTESIAN_POINT('',(4.75930776765241,-5.82847102381266E-16,10.8017566198263));
#3946=CARTESIAN_POINT('Origin',(0.,0.,14.3002821279377));
#3947=CARTESIAN_POINT('',(4.70116056230231,0.741687127224165,14.3002311117149));
#3948=CARTESIAN_POINT('Origin',(0.,0.,14.3002311117149));
#3949=CARTESIAN_POINT('',(4.70116056230231,0.741687127224165,7.30323111171487));
#3950=CARTESIAN_POINT('',(4.70116056230231,0.741687127224165,7.30323111171487));
#3951=CARTESIAN_POINT('Origin',(0.,0.,7.30323111171487));
#3952=CARTESIAN_POINT('Origin',(0.,0.,7.30323111171487));
#3953=CARTESIAN_POINT('Origin',(0.,0.,7.30323111171487));
#3954=CARTESIAN_POINT('Origin',(0.,0.,7.30323111171487));
#3955=CARTESIAN_POINT('Origin',(0.,0.,7.30323111171487));
#3956=CARTESIAN_POINT('Origin',(0.,0.,7.30323111171487));
#3957=CARTESIAN_POINT('Origin',(0.,0.,7.30323111171487));
#3958=CARTESIAN_POINT('Origin',(0.,0.,7.30323111171487));
#3959=CARTESIAN_POINT('Origin',(0.,0.,7.30323111171487));
#3960=CARTESIAN_POINT('Origin',(0.,0.,7.30323111171487));
#3961=CARTESIAN_POINT('Origin',(0.,0.,7.30323111171487));
#3962=CARTESIAN_POINT('Origin',(0.,0.,7.30323111171487));
#3963=CARTESIAN_POINT('Origin',(0.,0.,7.30323111171487));
#3964=CARTESIAN_POINT('Origin',(0.,0.,7.30323111171487));
#3965=CARTESIAN_POINT('',(4.70116056230231,-0.741687127224166,7.30323111171487));
#3966=CARTESIAN_POINT('Origin',(0.,0.,7.30323111171487));
#3967=CARTESIAN_POINT('',(4.70116056230231,-0.741687127224166,7.30323111171487));
#3968=CARTESIAN_POINT('Origin',(4.63877465489478,-0.848888570088464,7.30323111171487));
#3969=CARTESIAN_POINT('',(4.66517787878367,-0.727698551673083,7.30323111171487));
#3970=CARTESIAN_POINT('Origin',(4.63877465489478,-0.848888570088464,7.30323111171487));
#3971=CARTESIAN_POINT('',(4.66517787878367,-0.727698551673083,14.3002311117149));
#3972=CARTESIAN_POINT('',(4.66517787878367,-0.727698551673083,7.30323111171487));
#3973=CARTESIAN_POINT('Origin',(4.63877465489478,-0.848888570088464,14.3002311117149));
#3974=CARTESIAN_POINT('Origin',(5.13999824000407,0.,14.3002311117149));
#3975=CARTESIAN_POINT('',(4.66517787878367,0.727698551673083,14.3002311117149));
#3976=CARTESIAN_POINT('Origin',(4.84271052295884,4.85722573273506E-16,14.3002311117149));
#3977=CARTESIAN_POINT('Origin',(4.63877465489478,0.848888570088464,14.3002311117149));
#3978=CARTESIAN_POINT('Origin',(4.84271052295884,4.85722573273506E-16,7.30323111171487));
#3979=CARTESIAN_POINT('',(4.66517787878367,0.727698551673083,7.30323111171487));
#3980=CARTESIAN_POINT('Origin',(4.84271052295884,4.85722573273506E-16,7.30323111171487));
#3981=CARTESIAN_POINT('',(4.66517787878367,0.727698551673083,7.30323111171487));
#3982=CARTESIAN_POINT('Origin',(4.63877465489478,0.848888570088464,7.30323111171487));
#3983=CARTESIAN_POINT('Origin',(4.63877465489478,0.848888570088464,7.30323111171487));
#3984=CARTESIAN_POINT('Origin',(-4.75930776765241,0.,14.3002821279377));
#3985=CARTESIAN_POINT('',(6.71146155382814,-8.21916990949615E-16,14.3002821279377));
#3986=CARTESIAN_POINT('Origin',(0.,0.,14.3002821279377));
#3987=CARTESIAN_POINT('Origin',(-6.71146155382814,0.,7.30323111171487));
#3988=CARTESIAN_POINT('',(6.71146155382814,-8.21916990949615E-16,7.30323111171487));
#3989=CARTESIAN_POINT('Origin',(0.,0.,7.30323111171487));
#3990=CARTESIAN_POINT('Origin',(0.,0.,7.18611620816211));
#3991=CARTESIAN_POINT('',(6.94701057265674,-8.50763426144689E-16,7.06900130460935));
#3992=CARTESIAN_POINT('Origin',(0.,0.,7.06900130460935));
#3993=CARTESIAN_POINT('',(6.82923606324244,-8.36340208547153E-16,7.18611620816211));
#3994=CARTESIAN_POINT('Origin',(0.,0.,3.65014826262535));
#3995=CARTESIAN_POINT('',(6.94701057265674,-8.50763426144689E-16,0.231295220641352));
#3996=CARTESIAN_POINT('Origin',(0.,0.,0.231295220641352));
#3997=CARTESIAN_POINT('',(6.94701057265674,-8.5076342614469E-16,3.65014826262535));
#3998=CARTESIAN_POINT('',(6.94701057265674,-8.5076342614469E-16,3.65014826262535));
#3999=CARTESIAN_POINT('Origin',(0.,0.,0.115647610320677));
#4000=CARTESIAN_POINT('',(6.71701073999059,-8.22596570256787E-16,5.20417042793042E-16));
#4001=CARTESIAN_POINT('',(6.83201065632366,8.36679998200738E-16,0.115647610320677));
#4002=CARTESIAN_POINT('Origin',(0.,0.,0.));
#4003=CARTESIAN_POINT('Origin',(-4.88235460250674,0.,0.));
#4004=CARTESIAN_POINT('',(4.88235460250674,-5.97915993626222E-16,1.82145964977565E-16));
#4005=CARTESIAN_POINT('Origin',(0.,0.,0.));
#4006=CARTESIAN_POINT('Origin',(0.,0.,0.0596026238408975));
#4007=CARTESIAN_POINT('',(4.72357304027696,-5.78470860431392E-16,0.119205247681795));
#4008=CARTESIAN_POINT('Origin',(0.,0.,0.119205247681795));
#4009=CARTESIAN_POINT('',(4.80296382139185,-5.88193427028807E-16,0.0596026238408975));
#4010=CARTESIAN_POINT('Origin',(0.,0.,0.0596026238408975));
#4011=CARTESIAN_POINT('',(4.56686254190236,-5.59279359408668E-16,2.16840434497101E-16));
#4012=CARTESIAN_POINT('',(4.64521779108966,5.68875109920029E-16,0.0596026238408975));
#4013=CARTESIAN_POINT('Origin',(0.,0.,0.));
#4014=CARTESIAN_POINT('Origin',(-2.72176037385134,0.,0.));
#4015=CARTESIAN_POINT('',(2.72176037385134,-3.33319512988314E-16,-1.38777878078145E-16));
#4016=CARTESIAN_POINT('Origin',(0.,0.,0.));
#4017=CARTESIAN_POINT('Origin',(0.,0.,0.10956776965426));
#4018=CARTESIAN_POINT('',(2.61128051468949,-3.19789632399034E-16,0.10956776965426));
#4019=CARTESIAN_POINT('Origin',(0.,0.,15.3841467814851));
#4020=CARTESIAN_POINT('',(2.7303795503838,-3.34375057683491E-16,15.4998917859252));
#4021=CARTESIAN_POINT('',(2.61559010295572,3.20317404746622E-16,15.3841467814851));
#4022=CARTESIAN_POINT('Origin',(0.,0.,15.4998917859252));
#4023=CARTESIAN_POINT('Origin',(-4.56694754124435,0.,15.4998917859252));
#4024=CARTESIAN_POINT('',(4.56694754124434,-5.59289768825876E-16,15.4998917859252));
#4025=CARTESIAN_POINT('Origin',(0.,0.,15.4998917859252));
#4026=CARTESIAN_POINT('Origin',(0.,0.,15.4392892165051));
#4027=CARTESIAN_POINT('',(4.72346421955602,-5.78457533736633E-16,15.378686647085));
#4028=CARTESIAN_POINT('Origin',(0.,0.,15.378686647085));
#4029=CARTESIAN_POINT('',(4.64520588040018,-5.68873651281254E-16,15.4392892165051));
#4030=CARTESIAN_POINT('Origin',(0.,0.,15.4392892165051));
#4031=CARTESIAN_POINT('',(4.8865982268606,-5.98435687724396E-16,15.4998917859252));
#4032=CARTESIAN_POINT('',(4.80503122320831,5.88446610730515E-16,15.4392892165051));
#4033=CARTESIAN_POINT('Origin',(0.,0.,15.4998917859252));
#4034=CARTESIAN_POINT('Origin',(-6.72522523865914,0.,15.4998917859252));
#4035=CARTESIAN_POINT('',(6.72522523865914,-8.23602556206891E-16,15.4998917859252));
#4036=CARTESIAN_POINT('Origin',(0.,0.,15.4998917859252));
#4037=CARTESIAN_POINT('Origin',(0.,0.,15.3866394833227));
#4038=CARTESIAN_POINT('',(6.94665463816359,-8.50719836740916E-16,15.2733871807203));
#4039=CARTESIAN_POINT('Origin',(0.,0.,15.2733871807203));
#4040=CARTESIAN_POINT('',(6.83593993841137,-8.37161196473904E-16,15.3866394833227));
#4041=CARTESIAN_POINT('Origin',(0.,0.,14.9017962538623));
#4042=CARTESIAN_POINT('',(6.94665463816359,-8.50719836740916E-16,14.5302053270043));
#4043=CARTESIAN_POINT('Origin',(0.,0.,14.5302053270043));
#4044=CARTESIAN_POINT('',(6.94665463816359,-8.50719836740916E-16,14.9017962538623));
#4045=CARTESIAN_POINT('Origin',(0.,0.,14.415243727471));
#4046=CARTESIAN_POINT('',(6.82905809599587,8.36318413845266E-16,14.415243727471));
#12110=UNCERTAINTY_MEASURE_WITH_UNIT(LENGTH_MEASURE(0.01),#12119,
'DISTANCE_ACCURACY_VALUE',
'Maximum model space distance between geometric entities at asserted c
onnectivities');
#12113=UNCERTAINTY_MEASURE_WITH_UNIT(LENGTH_MEASURE(0.01),#12119,
'DISTANCE_ACCURACY_VALUE',
'Maximum model space distance between geometric entities at asserted c
onnectivities');
#12115=(
GEOMETRIC_REPRESENTATION_CONTEXT(3)
GLOBAL_UNCERTAINTY_ASSIGNED_CONTEXT((#12110))
GLOBAL_UNIT_ASSIGNED_CONTEXT((#12119,#12121,#12122))
REPRESENTATION_CONTEXT('','3D')
);
#12118=(
GEOMETRIC_REPRESENTATION_CONTEXT(3)
GLOBAL_UNCERTAINTY_ASSIGNED_CONTEXT((#12113))
GLOBAL_UNIT_ASSIGNED_CONTEXT((#12119,#12121,#12122))
REPRESENTATION_CONTEXT('','3D')
);
#12119=(
LENGTH_UNIT()
NAMED_UNIT(*)
SI_UNIT(.MILLI.,.METRE.)
);
#12121=(
NAMED_UNIT(*)
PLANE_ANGLE_UNIT()
SI_UNIT($,.RADIAN.)
);
#12122=(
NAMED_UNIT(*)
SI_UNIT($,.STERADIAN.)
SOLID_ANGLE_UNIT()
);
#12124=SHAPE_DEFINITION_REPRESENTATION(#12128,#12135);
#12128=PRODUCT_DEFINITION_SHAPE('',$,#12140);
#12135=SHAPE_REPRESENTATION('',(#2444),#12115);
#12138=PRODUCT_DEFINITION_CONTEXT('part definition',#12152,'design');
#12140=PRODUCT_DEFINITION('Pully','Pully',#12144,#12138);
#12144=PRODUCT_DEFINITION_FORMATION('',$,#12155);
#12152=APPLICATION_CONTEXT(
'Core Data for Automotive Mechanical Design Process');
#12153=PRODUCT_CONTEXT('part definition',#12152,'mechanical');
#12155=PRODUCT('Pully','Pully',$,(#12153));
#12159=PRESENTATION_STYLE_ASSIGNMENT((#12161));
#12161=SURFACE_STYLE_USAGE(.BOTH.,#12163);
#12163=SURFACE_SIDE_STYLE('',(#12165));
#12165=SURFACE_STYLE_FILL_AREA(#12167);
#12167=FILL_AREA_STYLE('Opaque(160,160,160)',(#12169));
#12169=FILL_AREA_STYLE_COLOUR('Opaque(160,160,160)',#12171);
#12171=COLOUR_RGB('Opaque(160,160,160)', 0.09019608, 0.27058824, 0.51372549);
ENDSEC;
END-ISO-10303-21;
